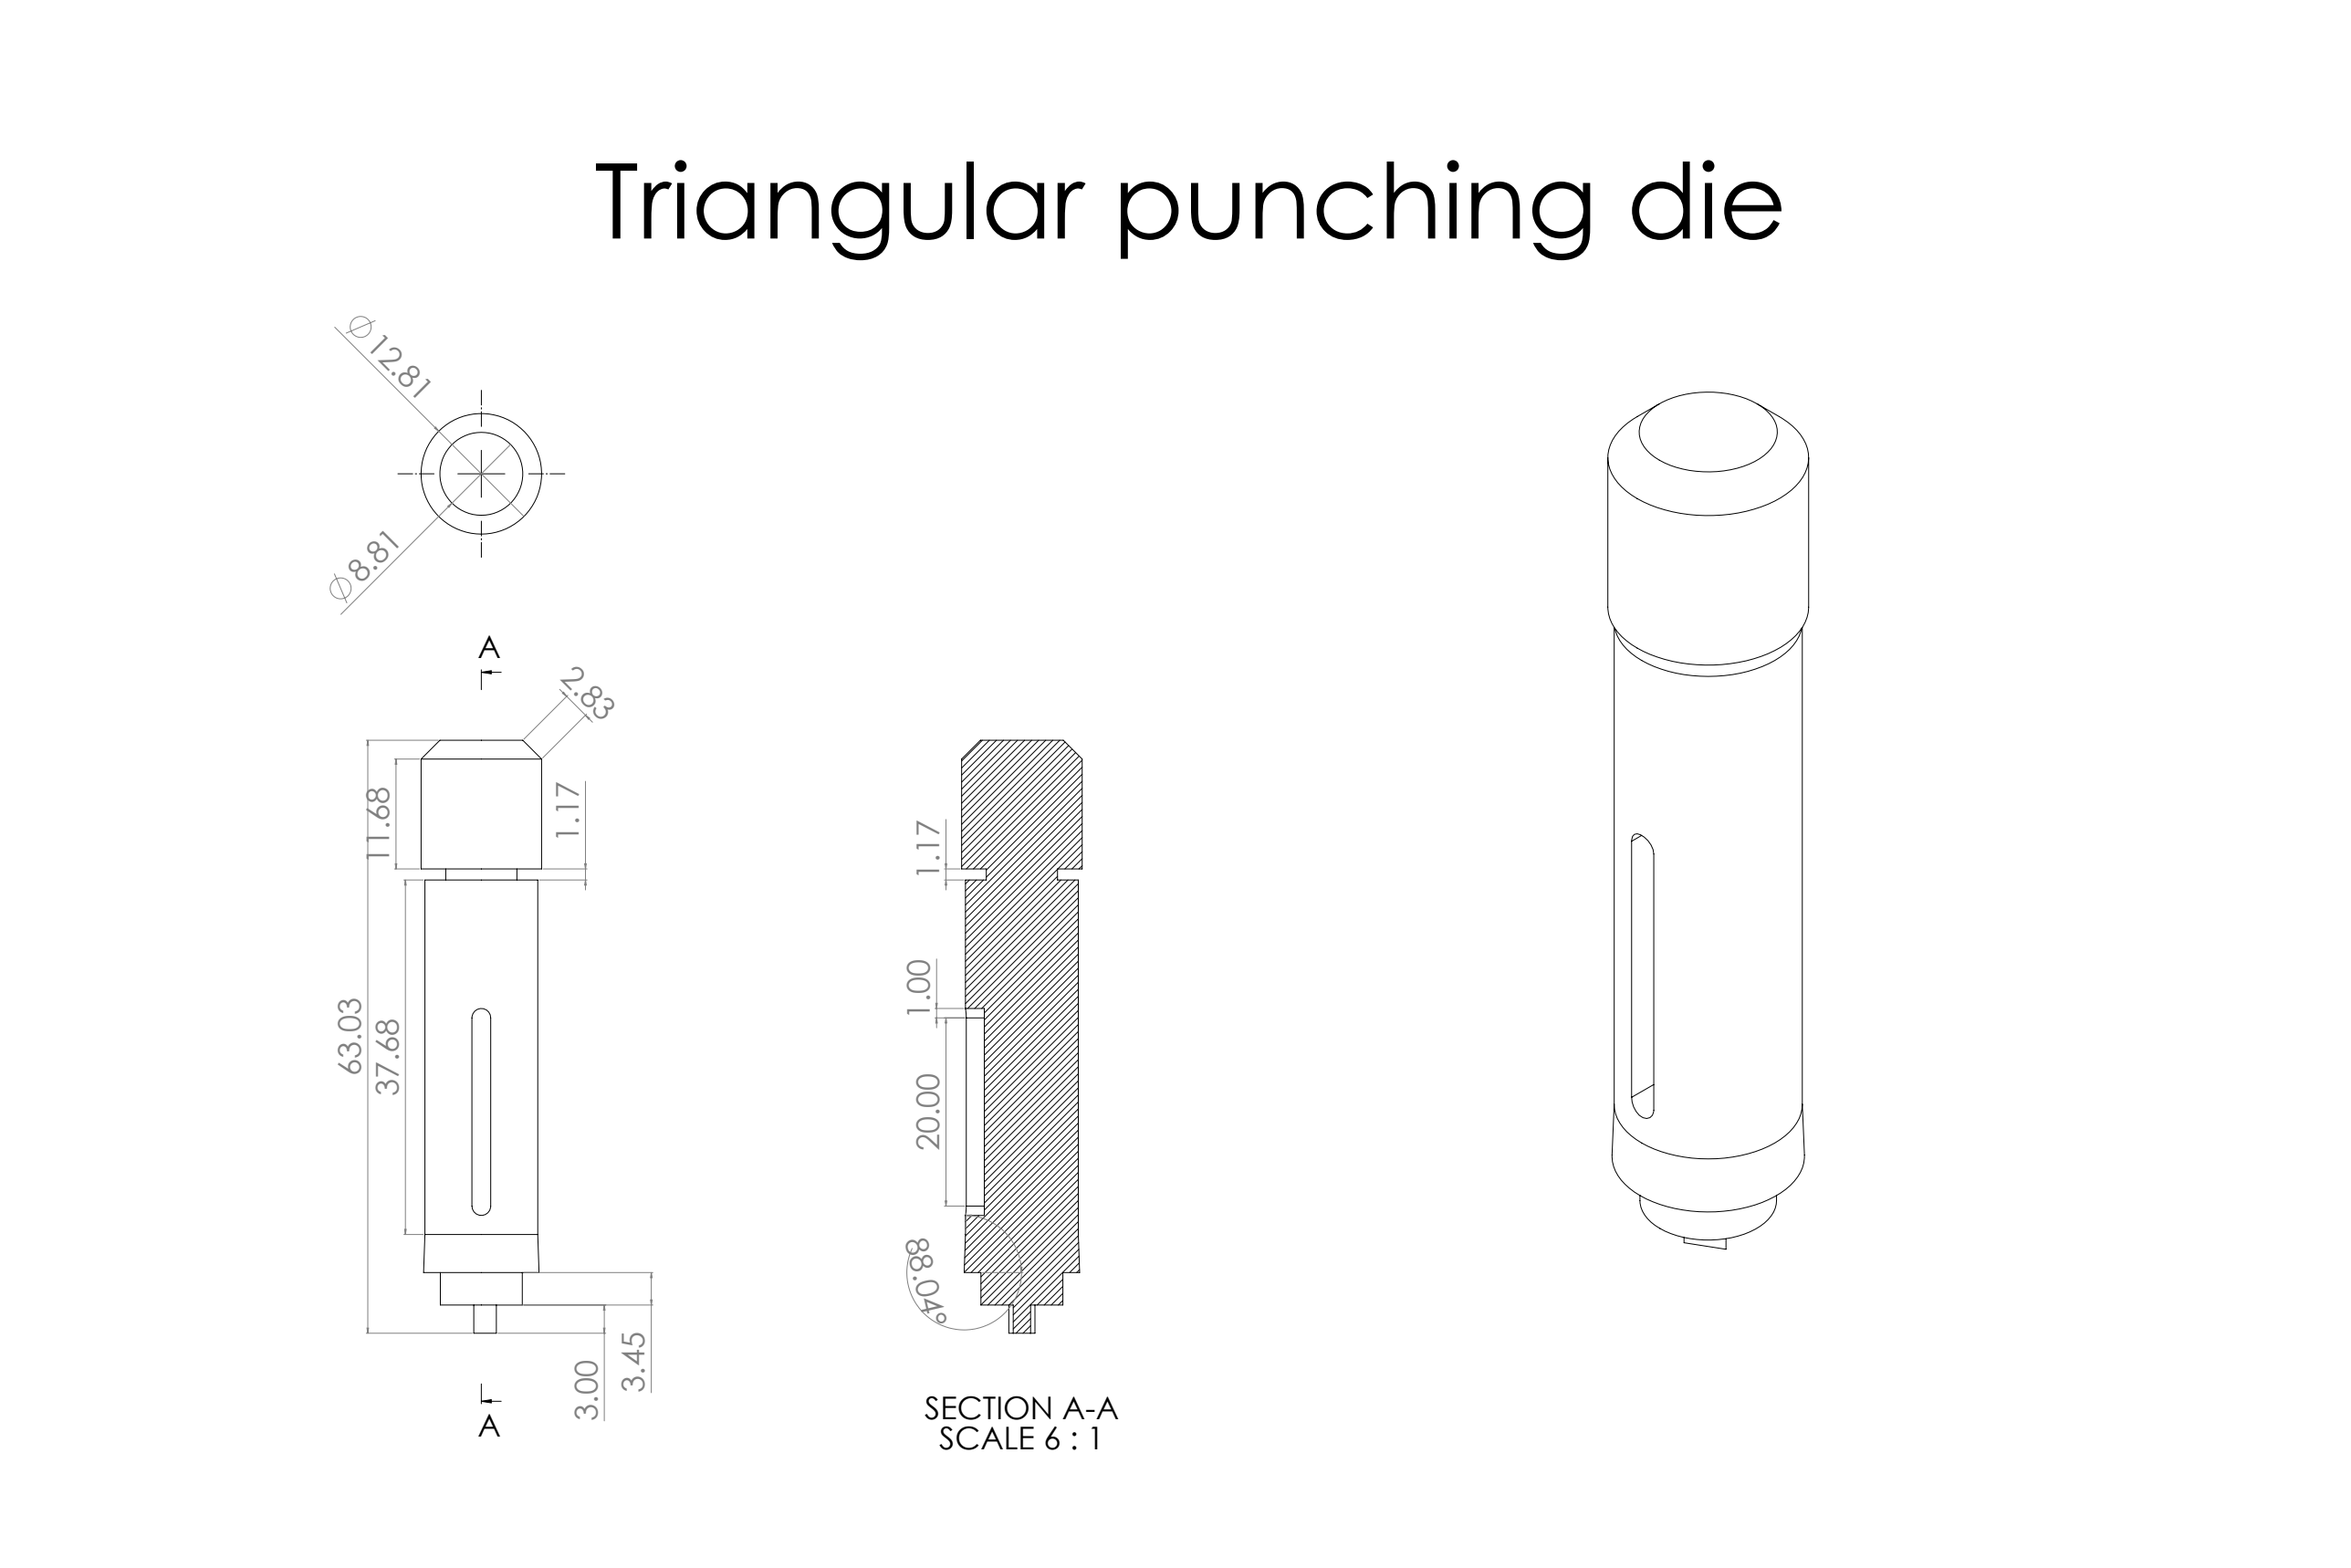
ISO-10303-21;
HEADER;
FILE_DESCRIPTION (('STEP AP214'),
    '1' );
FILE_NAME ('Triangular punching die.step',
    '2026-10-24T22:54:28',
    ( '' ),
    ( '' ),
    'SwSTEP 2.0',
    'SolidWorks 2025',
    '' );
FILE_SCHEMA (( 'AUTOMOTIVE_DESIGN' ));
ENDSEC;

DATA;
#6=DIRECTION ( 'NONE',  ( 0.000000000000000000, -1.000000000000000000, 0.000000000000000000 ) ) ;
#9=CARTESIAN_POINT ( 'NONE',  ( -69.92837670882107659, -20.78299143688747819, 3.916079783099623679 ) ) ;
#20=ORIENTED_EDGE ( 'NONE', *, *, #32884, .T. ) ;
#72=DIRECTION ( 'NONE',  ( -0.000000000000000000, 1.000000000000000000, -0.000000000000000000 ) ) ;
#76=EDGE_CURVE ( 'NONE', #14380, #23841, #36922, .T. ) ;
#84=DIRECTION ( 'NONE',  ( 0.8660254037844393737, 0.000000000000000000, 0.4999999999999985567 ) ) ;
#98=ORIENTED_EDGE ( 'NONE', *, *, #35067, .F. ) ;
#125=EDGE_CURVE ( 'NONE', #38679, #29790, #4804, .T. ) ;
#202=ORIENTED_EDGE ( 'NONE', *, *, #26812, .F. ) ;
#306=ORIENTED_EDGE ( 'NONE', *, *, #22254, .F. ) ;
#395=CIRCLE ( 'NONE', #29328, 6.406751979251626317 ) ;
#462=VERTEX_POINT ( 'NONE', #32769 ) ;
#473=CARTESIAN_POINT ( 'NONE',  ( -70.92837670882107659, 26.72470171467712063, 0.000000000000000000 ) ) ;
#571=ADVANCED_FACE ( 'NONE', ( #22696 ), #35460, .T. ) ;
#611=CARTESIAN_POINT ( 'NONE',  ( -71.90198294515647603, -0.5205283187954542479, 5.920697336060230853 ) ) ;
#644=FACE_OUTER_BOUND ( 'NONE', #40034, .T. ) ;
#810=LINE ( 'NONE', #13343, #16776 ) ;
#853=CARTESIAN_POINT ( 'NONE',  ( -70.92837670882107659, -27.85319909218681644, 0.000000000000000000 ) ) ;
#900=ORIENTED_EDGE ( 'NONE', *, *, #14039, .T. ) ;
#923=FACE_BOUND ( 'NONE', #15811, .T. ) ;
#955=CIRCLE ( 'NONE', #2272, 6.406751979251626317 ) ;
#962=ORIENTED_EDGE ( 'NONE', *, *, #2526, .F. ) ;
#1010=VERTEX_POINT ( 'NONE', #1619 ) ;
#1197=CARTESIAN_POINT ( 'NONE',  ( -71.72837670882105954, -31.30579396504363388, -1.385640646055078307 ) ) ;
#1304=ORIENTED_EDGE ( 'NONE', *, *, #8540, .T. ) ;
#1306=CARTESIAN_POINT ( 'NONE',  ( -70.39213229241123315, 0.06107131307206801335, 5.988032920670404380 ) ) ;
#1331=ADVANCED_FACE ( 'NONE', ( #20901 ), #9845, .T. ) ;
#1414=CARTESIAN_POINT ( 'NONE',  ( -71.78177034180626492, -21.31587262608876543, 5.951446729975963912 ) ) ;
#1470=DIRECTION ( 'NONE',  ( 0.000000000000000000, 0.000000000000000000, 1.000000000000000000 ) ) ;
#1495=CARTESIAN_POINT ( 'NONE',  ( -70.92837670882107659, 28.72470171467712063, 0.000000000000000000 ) ) ;
#1568=DIRECTION ( 'NONE',  ( -0.000000000000000000, 1.000000000000000000, -0.000000000000000000 ) ) ;
#1574=EDGE_LOOP ( 'NONE', ( #33274, #14393, #25939, #14553 ) ) ;
#1583=LINE ( 'NONE', #1197, #20933 ) ;
#1607=CARTESIAN_POINT ( 'NONE',  ( -71.92837670882107659, -20.78299143688747819, 5.928123921495630277 ) ) ;
#1615=EDGE_LOOP ( 'NONE', ( #22756, #962 ) ) ;
#1619=CARTESIAN_POINT ( 'NONE',  ( -70.92837670882107659, 28.72470171467712063, -4.406751979251624540 ) ) ;
#1643=CYLINDRICAL_SURFACE ( 'NONE', #6437, 6.406751979251626317 ) ;
#1676=CARTESIAN_POINT ( 'NONE',  ( -70.92837670882074974, 0.2169278855384722815, 6.000000000000007994 ) ) ;
#1704=CARTESIAN_POINT ( 'NONE',  ( -70.70332177653823180, 0.1913546399533780362, 3.995777704139396924 ) ) ;
#1788=DIRECTION ( 'NONE',  ( 0.8660254037844393737, 0.000000000000000000, 0.4999999999999985567 ) ) ;
#1814=CARTESIAN_POINT ( 'NONE',  ( -71.46462112523092003, -21.62705418684702252, 5.988032920670398163 ) ) ;
#1828=CARTESIAN_POINT ( 'NONE',  ( -70.42442292110172275, -21.65671257467926836, 5.980030958859729573 ) ) ;
#1962=DIRECTION ( 'NONE',  ( 1.000000000000000000, 0.000000000000000000, 0.000000000000000000 ) ) ;
#1987=ADVANCED_FACE ( 'NONE', ( #2899 ), #14440, .T. ) ;
#2112=CARTESIAN_POINT ( 'NONE',  ( -70.21272673770054951, -0.07566977545864603250, 3.957576123060443596 ) ) ;
#2119=CARTESIAN_POINT ( 'NONE',  ( -71.90228189594579078, -21.04538751579064737, 5.920650877785229582 ) ) ;
#2218=CARTESIAN_POINT ( 'NONE',  ( -69.92837670882107659, -20.78299143688747819, 5.928123921495640936 ) ) ;
#2272=AXIS2_PLACEMENT_3D ( 'NONE', #11107, #29658, #1470 ) ;
#2282=VERTEX_POINT ( 'NONE', #23335 ) ;
#2314=CARTESIAN_POINT ( 'NONE',  ( -71.70854571598145810, -0.1474806467180565794, 5.961650403247826802 ) ) ;
#2318=AXIS2_PLACEMENT_3D ( 'NONE', #30036, #14373, #26943 ) ;
#2319=ORIENTED_EDGE ( 'NONE', *, *, #33578, .T. ) ;
#2323=CARTESIAN_POINT ( 'NONE',  ( -71.54295603092448630, -21.58232592843834396, 5.969163363928941202 ) ) ;
#2365=DIRECTION ( 'NONE',  ( -0.000000000000000000, 1.000000000000000000, 0.000000000000000000 ) ) ;
#2370=CIRCLE ( 'NONE', #36523, 6.000000000000005329 ) ;
#2436=CARTESIAN_POINT ( 'NONE',  ( -70.30712919725708332, -21.57437711518543111, 5.980324962551068602 ) ) ;
#2496=CARTESIAN_POINT ( 'NONE',  ( -71.45033707005815415, -21.67496598542010489, 3.980161455544446891 ) ) ;
#2526=EDGE_CURVE ( 'NONE', #5538, #38785, #4624, .T. ) ;
#2543=ORIENTED_EDGE ( 'NONE', *, *, #24789, .T. ) ;
#2557=AXIS2_PLACEMENT_3D ( 'NONE', #15181, #27740, #40293 ) ;
#2563=LINE ( 'NONE', #40201, #30748 ) ;
#2576=CIRCLE ( 'NONE', #38044, 4.357836081054403010 ) ;
#2617=CARTESIAN_POINT ( 'NONE',  ( -70.92837670882107659, -31.30579396504363388, 0.000000000000000000 ) ) ;
#2622=EDGE_CURVE ( 'NONE', #23841, #33142, #10877, .T. ) ;
#2731=CARTESIAN_POINT ( 'NONE',  ( -71.92837670882107659, -0.7434385580723641418, 3.916079783099621014 ) ) ;
#2824=VECTOR ( 'NONE', #17716, 1000.000000000000000 ) ;
#2844=CARTESIAN_POINT ( 'NONE',  ( -71.15343164110390717, -21.75733751372833069, 6.007821842535416401 ) ) ;
#2862=EDGE_CURVE ( 'NONE', #1010, #27757, #28317, .T. ) ;
#2899=FACE_OUTER_BOUND ( 'NONE', #9131, .T. ) ;
#2934=B_SPLINE_CURVE_WITH_KNOTS ( 'NONE', 3,
 ( #8373, #17839, #39671, #1828, #26919, #27121, #5304, #39463, #11454, #23815 ),
 .UNSPECIFIED., .F., .F.,
 ( 4, 2, 2, 2, 4 ),
 ( 0.001566344281586717164, 0.001957551653609773592, 0.002348759025632830236, 0.002739966397655886447, 0.003131173769678943092 ),
 .UNSPECIFIED. ) ;
#2950=DIRECTION ( 'NONE',  ( -0.000000000000000000, 1.000000000000000000, -0.000000000000000000 ) ) ;
#3016=VECTOR ( 'NONE', #6358, 1000.000000000000000 ) ;
#3038=CARTESIAN_POINT ( 'NONE',  ( -69.95453796102918886, -0.5206348589351952327, 3.920659437262051128 ) ) ;
#3059=CARTESIAN_POINT ( 'NONE',  ( -71.26311553261176357, -21.73200267494512161, 3.991660656778087901 ) ) ;
#3150=CARTESIAN_POINT ( 'NONE',  ( -70.92661119047551210, 0.2232129446074198609, 6.013069300985390164 ) ) ;
#3160=FACE_OUTER_BOUND ( 'NONE', #26573, .T. ) ;
#3178=ORIENTED_EDGE ( 'NONE', *, *, #7572, .F. ) ;
#3212=ADVANCED_FACE ( 'NONE', ( #20406 ), #22912, .F. ) ;
#3215=CYLINDRICAL_SURFACE ( 'NONE', #32680, 6.000000000000005329 ) ;
#3394=CARTESIAN_POINT ( 'NONE',  ( -71.92837670882107659, -0.7829914368874776320, 3.916079783099624567 ) ) ;
#3430=CARTESIAN_POINT ( 'NONE',  ( -70.92837670882107659, -27.85319909218681644, 0.000000000000000000 ) ) ;
#3553=DIRECTION ( 'NONE',  ( 1.000000000000000000, 0.000000000000000000, 0.000000000000000000 ) ) ;
#3556=VERTEX_POINT ( 'NONE', #37877 ) ;
#3634=AXIS2_PLACEMENT_3D ( 'NONE', #8388, #17438, #33545 ) ;
#3739=DIRECTION ( 'NONE',  ( 0.000000000000000000, 0.000000000000000000, 1.000000000000000000 ) ) ;
#3782=DIRECTION ( 'NONE',  ( 0.000000000000000000, 0.000000000000000000, -1.000000000000000000 ) ) ;
#3794=PLANE ( 'NONE',  #7689 ) ;
#3809=AXIS2_PLACEMENT_3D ( 'NONE', #18051, #21163, #14976 ) ;
#3859=ORIENTED_EDGE ( 'NONE', *, *, #10125, .F. ) ;
#3874=AXIS2_PLACEMENT_3D ( 'NONE', #7544, #7343, #4273 ) ;
#3898=EDGE_CURVE ( 'NONE', #16025, #29790, #6157, .T. ) ;
#3957=VECTOR ( 'NONE', #1568, 1000.000000000000000 ) ;
#3959=B_SPLINE_CURVE_WITH_KNOTS ( 'NONE', 3,
 ( #34198, #37249, #8629, #33779, #5557, #2496, #33990, #24286 ),
 .UNSPECIFIED., .F., .F.,
 ( 4, 2, 2, 4 ),
 ( 0.000000000000000000, 0.1250305178534004968, 0.2500610357068009937, 0.5001220714135948819 ),
 .UNSPECIFIED. ) ;
#3972=CARTESIAN_POINT ( 'NONE',  ( -70.12941285977503014, -0.1676659666690925865, 5.947291465561957757 ) ) ;
#4011=VERTEX_POINT ( 'NONE', #4097 ) ;
#4055=SHAPE_DEFINITION_REPRESENTATION ( #35129, #39290 ) ;
#4058=EDGE_CURVE ( 'NONE', #25957, #16025, #11437, .T. ) ;
#4097=CARTESIAN_POINT ( 'NONE',  ( -70.92837670882107659, -23.80776546975053165, 6.000000000000005329 ) ) ;
#4138=ORIENTED_EDGE ( 'NONE', *, *, #11281, .F. ) ;
#4201=CARTESIAN_POINT ( 'NONE',  ( -71.72837670882105954, -34.30579396504363388, 1.385640646055090519 ) ) ;
#4229=PRODUCT ( 'Triangular punching die', 'Triangular punching die', '', ( #32256 ) ) ;
#4233=PLANE ( 'NONE',  #15168 ) ;
#4273=DIRECTION ( 'NONE',  ( 0.000000000000000000, 0.000000000000000000, 1.000000000000000000 ) ) ;
#4395=CARTESIAN_POINT ( 'NONE',  ( -69.92837670882107659, -0.6719362264620037939, 5.928123921495636495 ) ) ;
#4483=CARTESIAN_POINT ( 'NONE',  ( 0.000000000000000000, -34.30579396504363388, 0.000000000000000000 ) ) ;
#4501=CARTESIAN_POINT ( 'NONE',  ( -71.90933819610624766, -21.00662979218648374, 3.919381273429904056 ) ) ;
#4624=CIRCLE ( 'NONE', #20378, 6.138794830819693793 ) ;
#4660=EDGE_CURVE ( 'NONE', #5702, #13186, #26402, .T. ) ;
#4688=CARTESIAN_POINT ( 'NONE',  ( -71.64402667994158946, -21.49031309831630665, 5.969620261456463517 ) ) ;
#4775=CARTESIAN_POINT ( 'NONE',  ( -70.14355411941724583, -0.1632709328201389365, 5.960493810635122180 ) ) ;
#4804=B_SPLINE_CURVE_WITH_KNOTS ( 'NONE', 3,
 ( #11778, #5840, #36316, #5020, #14672, #36713, #8496, #6456, #34681, #3394 ),
 .UNSPECIFIED., .F., .F.,
 ( 4, 2, 2, 2, 4 ),
 ( 0.5001220714136037637, 0.6250915535602028505, 0.7500610357068019374, 0.8750305178534010242, 1.000000000000000000 ),
 .UNSPECIFIED. ) ;
#4915=FACE_OUTER_BOUND ( 'NONE', #7970, .T. ) ;
#4923=VERTEX_POINT ( 'NONE', #39919 ) ;
#4937=( LENGTH_UNIT ( ) NAMED_UNIT ( * ) SI_UNIT ( .MILLI., .METRE. ) );
#5016=AXIS2_PLACEMENT_3D ( 'NONE', #35112, #28916, #32018 ) ;
#5020=CARTESIAN_POINT ( 'NONE',  ( -71.43157283993535600, 0.09103159405784894131, 3.980077070333584821 ) ) ;
#5066=DIRECTION ( 'NONE',  ( 0.000000000000000000, 0.000000000000000000, 1.000000000000000000 ) ) ;
#5088=CARTESIAN_POINT ( 'NONE',  ( -71.83651116356016075, -21.21610000639230975, 3.930990725878106495 ) ) ;
#5098=VECTOR ( 'NONE', #39151, 1000.000000000000000 ) ;
#5170=EDGE_CURVE ( 'NONE', #10250, #36751, #27655, .T. ) ;
#5227=PLANE ( 'NONE',  #5811 ) ;
#5275=ORIENTED_EDGE ( 'NONE', *, *, #7116, .F. ) ;
#5281=ORIENTED_EDGE ( 'NONE', *, *, #38674, .T. ) ;
#5304=CARTESIAN_POINT ( 'NONE',  ( -70.05487543777402948, -21.28726014413347656, 5.936291904728155266 ) ) ;
#5317=VERTEX_POINT ( 'NONE', #21005 ) ;
#5385=CARTESIAN_POINT ( 'NONE',  ( -71.92602134074772380, -0.7038144147489171498, 3.916479336966925295 ) ) ;
#5426=DIRECTION ( 'NONE',  ( -0.000000000000000000, 1.000000000000000000, -0.000000000000000000 ) ) ;
#5476=CARTESIAN_POINT ( 'NONE',  ( -69.32837670882108227, -31.30579396504363388, 1.870248747537495149E-15 ) ) ;
#5493=CARTESIAN_POINT ( 'NONE',  ( -70.03118149891237465, -21.22462562410226994, 5.944584973090443647 ) ) ;
#5538=VERTEX_POINT ( 'NONE', #40533 ) ;
#5557=CARTESIAN_POINT ( 'NONE',  ( -71.72810306468316810, -21.39745238146776884, 3.947195235487914289 ) ) ;
#5702=VERTEX_POINT ( 'NONE', #29808 ) ;
#5703=CARTESIAN_POINT ( 'NONE',  ( -69.92837670882107659, -20.82254431570259001, 5.928123921495640936 ) ) ;
#5710=VERTEX_POINT ( 'NONE', #16834 ) ;
#5712=AXIS2_PLACEMENT_3D ( 'NONE', #30670, #9024, #24268 ) ;
#5807=CARTESIAN_POINT ( 'NONE',  ( -71.92837670882107659, -20.78299143688747819, 5.916079783099621459 ) ) ;
#5811=AXIS2_PLACEMENT_3D ( 'NONE', #18177, #2365, #9122 ) ;
#5840=CARTESIAN_POINT ( 'NONE',  ( -71.06003735762037365, 0.2170295740194823630, 3.999999999923639304 ) ) ;
#5870=EDGE_LOOP ( 'NONE', ( #27582, #40559, #22660, #20284 ) ) ;
#5893=DIRECTION ( 'NONE',  ( 4.199171463528975886E-18, -0.9994119649315837961, 0.03428883712799970368 ) ) ;
#5988=EDGE_LOOP ( 'NONE', ( #30833, #13755, #27770, #37888 ) ) ;
#6023=DIRECTION ( 'NONE',  ( -0.000000000000000000, 1.000000000000000000, -0.000000000000000000 ) ) ;
#6116=CARTESIAN_POINT ( 'NONE',  ( -70.81922763566456069, -21.77701682883130019, 6.011051262898291725 ) ) ;
#6142=EDGE_CURVE ( 'NONE', #4923, #5702, #21778, .T. ) ;
#6157=LINE ( 'NONE', #31279, #12541 ) ;
#6271=ORIENTED_EDGE ( 'NONE', *, *, #11072, .T. ) ;
#6358=DIRECTION ( 'NONE',  ( 0.000000000000000000, 0.000000000000000000, -1.000000000000000000 ) ) ;
#6427=CARTESIAN_POINT ( 'NONE',  ( -70.31344945295795412, -21.58221595790078950, 3.969121680884525105 ) ) ;
#6437=AXIS2_PLACEMENT_3D ( 'NONE', #10485, #14181, #23065 ) ;
#6456=CARTESIAN_POINT ( 'NONE',  ( -71.90176653367559823, -0.5198039855910460139, 3.920732911925276287 ) ) ;
#6490=ORIENTED_EDGE ( 'NONE', *, *, #4660, .F. ) ;
#6630=EDGE_CURVE ( 'NONE', #38785, #5538, #36078, .T. ) ;
#6719=EDGE_CURVE ( 'NONE', #39731, #33142, #10570, .T. ) ;
#6822=DIRECTION ( 'NONE',  ( -0.000000000000000000, 1.000000000000000000, -0.000000000000000000 ) ) ;
#6930=LINE ( 'NONE', #11967, #25648 ) ;
#6931=ORIENTED_EDGE ( 'NONE', *, *, #33578, .F. ) ;
#6990=VERTEX_POINT ( 'NONE', #25378 ) ;
#7031=CARTESIAN_POINT ( 'NONE',  ( -70.05520034786580652, -0.2785546670064985575, 5.936342406970505969 ) ) ;
#7083=VERTEX_POINT ( 'NONE', #36807 ) ;
#7111=CARTESIAN_POINT ( 'NONE',  ( -70.92837670882107659, 28.72470171467712063, 6.000000000000005329 ) ) ;
#7116=EDGE_CURVE ( 'NONE', #6990, #34705, #20268, .T. ) ;
#7126=ORIENTED_EDGE ( 'NONE', *, *, #39294, .T. ) ;
#7232=CARTESIAN_POINT ( 'NONE',  ( -70.92837670882107659, 28.72470171467712063, -2.000000000000000000 ) ) ;
#7233=CARTESIAN_POINT ( 'NONE',  ( -69.92837670882107659, -0.6505659821428084744, 5.916079783099619682 ) ) ;
#7254=DIRECTION ( 'NONE',  ( 0.000000000000000000, 0.000000000000000000, 1.000000000000000000 ) ) ;
#7276=ORIENTED_EDGE ( 'NONE', *, *, #11043, .T. ) ;
#7343=DIRECTION ( 'NONE',  ( -0.000000000000000000, 1.000000000000000000, -0.000000000000000000 ) ) ;
#7357=B_SPLINE_CURVE_WITH_KNOTS ( 'NONE', 3,
 ( #8551, #8957, #3038, #14721, #24414, #34122, #18021, #11630 ),
 .UNSPECIFIED., .F., .F.,
 ( 4, 2, 2, 4 ),
 ( 0.000000000000000000, 0.1250305178534032724, 0.2500610357068065448, 0.5001220714136037637 ),
 .UNSPECIFIED. ) ;
#7367=CARTESIAN_POINT ( 'NONE',  ( -71.26311553261176357, -21.73200267494512161, 6.003704795174108710 ) ) ;
#7423=CARTESIAN_POINT ( 'NONE',  ( -69.92837670882107659, -20.78299143688747819, 5.916079783099620570 ) ) ;
#7434=FACE_BOUND ( 'NONE', #33299, .T. ) ;
#7486=FACE_OUTER_BOUND ( 'NONE', #22537, .T. ) ;
#7509=CIRCLE ( 'NONE', #35800, 4.406751979251624540 ) ;
#7544=CARTESIAN_POINT ( 'NONE',  ( -70.92837670882107659, -23.80776546975053165, 0.000000000000000000 ) ) ;
#7567=ORIENTED_EDGE ( 'NONE', *, *, #24444, .F. ) ;
#7572=EDGE_CURVE ( 'NONE', #10043, #14380, #28058, .T. ) ;
#7634=CARTESIAN_POINT ( 'NONE',  ( -69.92837670882107659, -0.7829914368874778541, 5.916079783099621459 ) ) ;
#7689=AXIS2_PLACEMENT_3D ( 'NONE', #16316, #32392, #28886 ) ;
#7767=AXIS2_PLACEMENT_3D ( 'NONE', #2617, #40052, #15341 ) ;
#7769=CARTESIAN_POINT ( 'NONE',  ( -71.78177034180626492, -21.31587262608876543, 3.939402591579943547 ) ) ;
#7809=AXIS2_PLACEMENT_3D ( 'NONE', #7232, #20184, #9916 ) ;
#7842=CARTESIAN_POINT ( 'NONE',  ( -64.92837670882106238, 13.87661300689593880, 0.000000000000000000 ) ) ;
#7858=DIRECTION ( 'NONE',  ( -0.000000000000000000, 1.000000000000000000, -0.000000000000000000 ) ) ;
#7874=CARTESIAN_POINT ( 'NONE',  ( -69.32837670882108227, -34.30579396504363388, 1.870248747537495149E-15 ) ) ;
#7970=EDGE_LOOP ( 'NONE', ( #19165, #8346, #10889, #5275 ) ) ;
#8049=FACE_OUTER_BOUND ( 'NONE', #12714, .T. ) ;
#8074=EDGE_CURVE ( 'NONE', #1010, #8622, #31565, .T. ) ;
#8105=EDGE_CURVE ( 'NONE', #34705, #6990, #32880, .T. ) ;
#8259=EDGE_LOOP ( 'NONE', ( #36223, #39781, #8815, #24678 ) ) ;
#8310=VECTOR ( 'NONE', #30487, 1000.000000000000000 ) ;
#8346=ORIENTED_EDGE ( 'NONE', *, *, #10125, .T. ) ;
#8350=EDGE_LOOP ( 'NONE', ( #10985, #31039, #38270 ) ) ;
#8373=CARTESIAN_POINT ( 'NONE',  ( -70.92837670882140344, -21.78291075931342391, 6.000000000000002665 ) ) ;
#8388=CARTESIAN_POINT ( 'NONE',  ( -71.72837670882105954, -34.30579396504363388, -1.385640646055078307 ) ) ;
#8390=DIRECTION ( 'NONE',  ( 0.000000000000000000, 0.000000000000000000, 1.000000000000000000 ) ) ;
#8440=VERTEX_POINT ( 'NONE', #38010 ) ;
#8448=DIRECTION ( 'NONE',  ( 0.000000000000000000, -1.000000000000000000, 0.000000000000000000 ) ) ;
#8454=CARTESIAN_POINT ( 'NONE',  ( -71.25654746924473670, 0.1680418597759353594, 6.003896035474988402 ) ) ;
#8496=CARTESIAN_POINT ( 'NONE',  ( -71.80166262301922586, -0.2784082907551633790, 3.936323582618165950 ) ) ;
#8540=EDGE_CURVE ( 'NONE', #39825, #5317, #6930, .T. ) ;
#8551=CARTESIAN_POINT ( 'NONE',  ( -69.92837670882107659, -0.7829914368874778541, 3.916079783099621014 ) ) ;
#8568=CARTESIAN_POINT ( 'NONE',  ( -70.70940173728274658, -21.76495738335424690, 6.009053033063224802 ) ) ;
#8570=EDGE_CURVE ( 'NONE', #23332, #27757, #40379, .T. ) ;
#8586=LINE ( 'NONE', #9350, #31786 ) ;
#8606=AXIS2_PLACEMENT_3D ( 'NONE', #34871, #72, #30754 ) ;
#8622=VERTEX_POINT ( 'NONE', #36346 ) ;
#8629=CARTESIAN_POINT ( 'NONE',  ( -71.90221545680498139, -21.04534801433412028, 3.920659437232132394 ) ) ;
#8647=DIRECTION ( 'NONE',  ( 0.000000000000000000, 0.000000000000000000, 1.000000000000000000 ) ) ;
#8659=CARTESIAN_POINT ( 'NONE',  ( -71.62860729996657483, -0.06907469158448548141, 3.958999674376896039 ) ) ;
#8666=CARTESIAN_POINT ( 'NONE',  ( -71.92837670882107659, -20.78299143688747819, 5.916079783099621459 ) ) ;
#8721=CARTESIAN_POINT ( 'NONE',  ( -69.92837670882107659, -20.78299143688747819, 5.916079783099621459 ) ) ;
#8764=ORIENTED_EDGE ( 'NONE', *, *, #11281, .T. ) ;
#8768=CARTESIAN_POINT ( 'NONE',  ( -69.93541594206888590, -20.90143516061696616, 3.917265324091089518 ) ) ;
#8815=ORIENTED_EDGE ( 'NONE', *, *, #25812, .F. ) ;
#8901=DIRECTION ( 'NONE',  ( -0.000000000000000000, 1.000000000000000000, -0.000000000000000000 ) ) ;
#8941=AXIS2_PLACEMENT_3D ( 'NONE', #21020, #39951, #8647 ) ;
#8957=CARTESIAN_POINT ( 'NONE',  ( -69.92844875602597199, -0.6521111472992819902, 3.916091961299970059 ) ) ;
#8958=CARTESIAN_POINT ( 'NONE',  ( -70.92837670882107659, 28.72470171467712063, 0.000000000000000000 ) ) ;
#8978=CARTESIAN_POINT ( 'NONE',  ( -70.14820770166069508, -21.41850222705690143, 3.949606264851799775 ) ) ;
#9024=DIRECTION ( 'NONE',  ( -0.000000000000000000, 1.000000000000000000, -0.000000000000000000 ) ) ;
#9057=ORIENTED_EDGE ( 'NONE', *, *, #40617, .T. ) ;
#9075=CARTESIAN_POINT ( 'NONE',  ( -71.82557191872977853, -0.3413572496726843264, 3.932540834694423726 ) ) ;
#9082=CARTESIAN_POINT ( 'NONE',  ( -71.92837670882107659, -20.91541689163215523, 5.916079783099619682 ) ) ;
#9091=CIRCLE ( 'NONE', #7767, 4.357836081054403010 ) ;
#9122=DIRECTION ( 'NONE',  ( 0.000000000000000000, 0.000000000000000000, 1.000000000000000000 ) ) ;
#9131=EDGE_LOOP ( 'NONE', ( #10423, #7126, #11894, #34602 ) ) ;
#9180=DIRECTION ( 'NONE',  ( -0.000000000000000000, 1.000000000000000000, -0.000000000000000000 ) ) ;
#9188=CARTESIAN_POINT ( 'NONE',  ( -70.60020594839741648, -21.73402473355089271, 6.003896035474983073 ) ) ;
#9260=CIRCLE ( 'NONE', #8606, 4.357836081054403010 ) ;
#9274=CARTESIAN_POINT ( 'NONE',  ( -71.62860729996657483, -0.06907469158448548141, 5.971043812772921733 ) ) ;
#9276=EDGE_CURVE ( 'NONE', #36200, #38679, #7357, .T. ) ;
#9302=EDGE_CURVE ( 'NONE', #4011, #5538, #34527, .T. ) ;
#9350=CARTESIAN_POINT ( 'NONE',  ( -70.92837670882107659, 28.72470171467712063, -3.784187430299790211 ) ) ;
#9485=DIRECTION ( 'NONE',  ( 0.000000000000000000, 0.000000000000000000, 1.000000000000000000 ) ) ;
#9569=ORIENTED_EDGE ( 'NONE', *, *, #27926, .F. ) ;
#9618=ADVANCED_FACE ( 'NONE', ( #10587 ), #4233, .F. ) ;
#9648=CIRCLE ( 'NONE', #5712, 3.784187430299790211 ) ;
#9697=B_SPLINE_CURVE_WITH_KNOTS ( 'NONE', 3,
 ( #8666, #9082, #2119, #36886, #27812, #2323, #21245, #21660, #40365, #18139 ),
 .UNSPECIFIED., .F., .F.,
 ( 4, 2, 2, 2, 4 ),
 ( 0.000000000000000000, 0.0003915860703966792910, 0.0007831721407933585821, 0.001174758211190037819, 0.001566344281586717164 ),
 .UNSPECIFIED. ) ;
#9702=VERTEX_POINT ( 'NONE', #18389 ) ;
#9797=ORIENTED_EDGE ( 'NONE', *, *, #3898, .F. ) ;
#9818=DIRECTION ( 'NONE',  ( -0.000000000000000000, 1.000000000000000000, -0.000000000000000000 ) ) ;
#9845=CONICAL_SURFACE ( 'NONE', #21667, 6.406751979251626317, 0.7853981633974482790 ) ;
#9899=ORIENTED_EDGE ( 'NONE', *, *, #22254, .T. ) ;
#9900=ADVANCED_FACE ( 'NONE', ( #19217 ), #35683, .T. ) ;
#9916=DIRECTION ( 'NONE',  ( 0.000000000000000000, 0.000000000000000000, 1.000000000000000000 ) ) ;
#9921=AXIS2_PLACEMENT_3D ( 'NONE', #24520, #14625, #21233 ) ;
#10043=VERTEX_POINT ( 'NONE', #17307 ) ;
#10114=VECTOR ( 'NONE', #36242, 1000.000000000000000 ) ;
#10125=EDGE_CURVE ( 'NONE', #2282, #8440, #37505, .T. ) ;
#10250=VERTEX_POINT ( 'NONE', #24104 ) ;
#10285=DIRECTION ( 'NONE',  ( -0.000000000000000000, 1.000000000000000000, -0.000000000000000000 ) ) ;
#10327=CARTESIAN_POINT ( 'NONE',  ( -69.92837670882107659, -0.7829914368874777431, 5.916079783099621459 ) ) ;
#10338=DIRECTION ( 'NONE',  ( -0.000000000000000000, 1.000000000000000000, -0.000000000000000000 ) ) ;
#10406=DIRECTION ( 'NONE',  ( 0.000000000000000000, 0.000000000000000000, 1.000000000000000000 ) ) ;
#10423=ORIENTED_EDGE ( 'NONE', *, *, #21751, .F. ) ;
#10453=DIRECTION ( 'NONE',  ( 0.000000000000000000, -0.9994119649315837961, -0.03428883712799970368 ) ) ;
#10485=CARTESIAN_POINT ( 'NONE',  ( -70.92837670882107659, 28.72470171467712063, 0.000000000000000000 ) ) ;
#10499=( NAMED_UNIT ( * ) SI_UNIT ( $, .STERADIAN. ) SOLID_ANGLE_UNIT ( ) );
#10544=ORIENTED_EDGE ( 'NONE', *, *, #6630, .T. ) ;
#10548=LINE ( 'NONE', #13442, #5098 ) ;
#10570=LINE ( 'NONE', #16944, #26860 ) ;
#10587=FACE_OUTER_BOUND ( 'NONE', #26046, .T. ) ;
#10628=ORIENTED_EDGE ( 'NONE', *, *, #30089, .F. ) ;
#10715=DIRECTION ( 'NONE',  ( 0.000000000000000000, -0.000000000000000000, -1.000000000000000000 ) ) ;
#10727=DIRECTION ( 'NONE',  ( 0.000000000000000000, 0.000000000000000000, 1.000000000000000000 ) ) ;
#10748=FACE_OUTER_BOUND ( 'NONE', #5870, .T. ) ;
#10815=EDGE_CURVE ( 'NONE', #40423, #4923, #9260, .T. ) ;
#10823=DIRECTION ( 'NONE',  ( -0.000000000000000000, 1.000000000000000000, -0.000000000000000000 ) ) ;
#10877=LINE ( 'NONE', #5476, #21705 ) ;
#10888=ORIENTED_EDGE ( 'NONE', *, *, #35911, .F. ) ;
#10889=ORIENTED_EDGE ( 'NONE', *, *, #14799, .T. ) ;
#10939=CARTESIAN_POINT ( 'NONE',  ( -70.92837670882107659, 28.72470171467712063, 4.000000000000005329 ) ) ;
#10983=DIRECTION ( 'NONE',  ( 0.000000000000000000, 0.000000000000000000, -1.000000000000000000 ) ) ;
#10985=ORIENTED_EDGE ( 'NONE', *, *, #7572, .T. ) ;
#11000=DIRECTION ( 'NONE',  ( -0.000000000000000000, 1.000000000000000000, -0.000000000000000000 ) ) ;
#11030=CARTESIAN_POINT ( 'NONE',  ( -70.92837670882107659, -23.80776546975053165, 0.000000000000000000 ) ) ;
#11042=CARTESIAN_POINT ( 'NONE',  ( -71.55887904216392315, -21.56717086459383026, 3.967530720604706573 ) ) ;
#11043=EDGE_CURVE ( 'NONE', #3556, #23841, #1583, .T. ) ;
#11054=EDGE_CURVE ( 'NONE', #13186, #5702, #2576, .T. ) ;
#11069=PLANE ( 'NONE',  #3634 ) ;
#11072=EDGE_CURVE ( 'NONE', #4011, #39825, #34110, .T. ) ;
#11107=CARTESIAN_POINT ( 'NONE',  ( -70.92837670882107659, 15.04836564048558500, 0.000000000000000000 ) ) ;
#11114=CARTESIAN_POINT ( 'NONE',  ( -70.92837670882074974, 0.2169278855384722815, 6.000000000000007994 ) ) ;
#11137=CARTESIAN_POINT ( 'NONE',  ( -70.21272673770054951, -0.07566977545864603250, 5.969620261456469734 ) ) ;
#11149=ORIENTED_EDGE ( 'NONE', *, *, #8074, .T. ) ;
#11198=DIRECTION ( 'NONE',  ( 8.659560562354932858E-17, -0.7071067811865474617, 0.7071067811865474617 ) ) ;
#11242=ORIENTED_EDGE ( 'NONE', *, *, #2862, .T. ) ;
#11281=EDGE_CURVE ( 'NONE', #4923, #40423, #9091, .T. ) ;
#11296=ORIENTED_EDGE ( 'NONE', *, *, #32884, .F. ) ;
#11334=CARTESIAN_POINT ( 'NONE',  ( -69.94741522153590552, -0.5593530815884721896, 3.919381273429904944 ) ) ;
#11422=DIRECTION ( 'NONE',  ( -0.000000000000000000, 1.000000000000000000, -0.000000000000000000 ) ) ;
#11434=DIRECTION ( 'NONE',  ( -0.000000000000000000, 1.000000000000000000, -0.000000000000000000 ) ) ;
#11437=LINE ( 'NONE', #27105, #15839 ) ;
#11442=CARTESIAN_POINT ( 'NONE',  ( -71.36981149190343388, -21.68728802194536698, 5.996540489601002832 ) ) ;
#11454=CARTESIAN_POINT ( 'NONE',  ( -69.92837670882109080, -20.91528719346852583, 5.916079783099622347 ) ) ;
#11475=MECHANICAL_DESIGN_GEOMETRIC_PRESENTATION_REPRESENTATION('',(#31237),#12133);
#11533=CIRCLE ( 'NONE', #30618, 6.406751979251626317 ) ;
#11551=ADVANCED_FACE ( 'NONE', ( #29536, #11990 ), #5227, .F. ) ;
#11630=CARTESIAN_POINT ( 'NONE',  ( -70.92837671539291478, 0.2169278822316458022, 3.999987187540717137 ) ) ;
#11647=CARTESIAN_POINT ( 'NONE',  ( -71.04476776058896803, -21.78243674987466605, 3.999856464806923473 ) ) ;
#11721=EDGE_LOOP ( 'NONE', ( #19383, #15515, #12945, #31925 ) ) ;
#11737=CARTESIAN_POINT ( 'NONE',  ( -71.35621909400492768, 0.1208619214844364048, 5.996770606117012292 ) ) ;
#11778=CARTESIAN_POINT ( 'NONE',  ( -70.92837671539291478, 0.2169278822316458022, 3.999987187540717137 ) ) ;
#11825=APPLICATION_CONTEXT ( 'automotive_design' ) ;
#11832=EDGE_CURVE ( 'NONE', #36751, #462, #26262, .T. ) ;
#11856=CARTESIAN_POINT ( 'NONE',  ( -70.93014222716664108, -21.78919581838237463, 4.001025162589363582 ) ) ;
#11894=ORIENTED_EDGE ( 'NONE', *, *, #35615, .T. ) ;
#11921=ORIENTED_EDGE ( 'NONE', *, *, #9276, .T. ) ;
#11947=CARTESIAN_POINT ( 'NONE',  ( -71.14735168035940660, 0.1989745095792901375, 3.997008894667205769 ) ) ;
#11950=ORIENTED_EDGE ( 'NONE', *, *, #33196, .F. ) ;
#11967=CARTESIAN_POINT ( 'NONE',  ( -70.92837670882107659, 28.72470171467712063, -6.000000000000005329 ) ) ;
#11990=FACE_BOUND ( 'NONE', #21791, .T. ) ;
#12133=( GEOMETRIC_REPRESENTATION_CONTEXT ( 3 ) GLOBAL_UNCERTAINTY_ASSIGNED_CONTEXT ( ( #37395 ) ) GLOBAL_UNIT_ASSIGNED_CONTEXT ( ( #23354, #25840, #32429 ) ) REPRESENTATION_CONTEXT ( 'NONE', 'WORKASPACE' ) );
#12166=ADVANCED_FACE ( 'NONE', ( #27197 ), #39755, .F. ) ;
#12327=MANIFOLD_SOLID_BREP ( 'Boss-Extrude8', #12401 ) ;
#12401=CLOSED_SHELL ( 'NONE', ( #39691, #1987, #25949, #21027, #39842, #35251, #13945, #36039, #9900, #12166, #13085, #28260, #37481, #27739, #13394, #11551, #29530, #1331, #38039, #26954, #37778, #38983, #571, #20533, #3212, #9618, #37540 ) ) ;
#12541=VECTOR ( 'NONE', #28168, 1000.000000000000000 ) ;
#12676=CARTESIAN_POINT ( 'NONE',  ( -70.92837670882107659, 28.72470171467712063, 0.000000000000000000 ) ) ;
#12714=EDGE_LOOP ( 'NONE', ( #37433, #13169, #24068, #21564, #13752, #13002 ) ) ;
#12720=DIRECTION ( 'NONE',  ( 0.000000000000000000, 0.000000000000000000, -1.000000000000000000 ) ) ;
#12721=LINE ( 'NONE', #37423, #3016 ) ;
#12737=CARTESIAN_POINT ( 'NONE',  ( -71.80187797986816634, -0.2787227296414631073, 5.936291904728147273 ) ) ;
#12767=ORIENTED_EDGE ( 'NONE', *, *, #4660, .T. ) ;
#12945=ORIENTED_EDGE ( 'NONE', *, *, #26812, .T. ) ;
#13002=ORIENTED_EDGE ( 'NONE', *, *, #125, .F. ) ;
#13052=AXIS2_PLACEMENT_3D ( 'NONE', #3430, #15942, #34919 ) ;
#13085=ADVANCED_FACE ( 'NONE', ( #644 ), #35029, .T. ) ;
#13169=ORIENTED_EDGE ( 'NONE', *, *, #35846, .F. ) ;
#13186=VERTEX_POINT ( 'NONE', #13788 ) ;
#13211=AXIS2_PLACEMENT_3D ( 'NONE', #1495, #7858, #7254 ) ;
#13343=CARTESIAN_POINT ( 'NONE',  ( -70.92837670882107659, -27.85319909218681644, -6.138794830819693793 ) ) ;
#13376=VECTOR ( 'NONE', #28065, 1000.000000000000000 ) ;
#13379=EDGE_LOOP ( 'NONE', ( #11149, #13464 ) ) ;
#13394=ADVANCED_FACE ( 'NONE', ( #4915 ), #17446, .T. ) ;
#13442=CARTESIAN_POINT ( 'NONE',  ( -70.92837670882107659, 28.72470171467712063, -4.357836081054403010 ) ) ;
#13464=ORIENTED_EDGE ( 'NONE', *, *, #21751, .T. ) ;
#13488=EDGE_CURVE ( 'NONE', #39731, #10043, #12721, .T. ) ;
#13536=VECTOR ( 'NONE', #3782, 1000.000000000000000 ) ;
#13611=CARTESIAN_POINT ( 'NONE',  ( -70.66586135525236045, 0.1905911290138092018, 5.995467141624639673 ) ) ;
#13707=ORIENTED_EDGE ( 'NONE', *, *, #20042, .F. ) ;
#13708=CARTESIAN_POINT ( 'NONE',  ( -70.92837670882107659, 26.72470171467712063, 6.406751979251626317 ) ) ;
#13752=ORIENTED_EDGE ( 'NONE', *, *, #3898, .T. ) ;
#13755=ORIENTED_EDGE ( 'NONE', *, *, #26456, .T. ) ;
#13772=VECTOR ( 'NONE', #84, 1000.000000000000114 ) ;
#13788=CARTESIAN_POINT ( 'NONE',  ( -70.92837670882107659, -27.85319909218681644, -4.357836081054403010 ) ) ;
#13804=( NAMED_UNIT ( * ) PLANE_ANGLE_UNIT ( ) SI_UNIT ( $, .RADIAN. ) );
#13852=EDGE_CURVE ( 'NONE', #27757, #30983, #11533, .T. ) ;
#13945=ADVANCED_FACE ( 'NONE', ( #28115 ), #18635, .T. ) ;
#14039=EDGE_CURVE ( 'NONE', #462, #5317, #15497, .T. ) ;
#14046=CARTESIAN_POINT ( 'NONE',  ( -70.92837670882107659, 28.72470171467712063, -2.000000000000000000 ) ) ;
#14127=AXIS2_PLACEMENT_3D ( 'NONE', #23261, #10285, #3739 ) ;
#14141=CARTESIAN_POINT ( 'NONE',  ( -71.64402667994158946, -21.49031309831630665, 3.957576123060442708 ) ) ;
#14181=DIRECTION ( 'NONE',  ( -0.000000000000000000, 1.000000000000000000, -0.000000000000000000 ) ) ;
#14235=CARTESIAN_POINT ( 'NONE',  ( -70.81198565705318515, 0.2164538760997103128, 6.011900603202949611 ) ) ;
#14369=AXIS2_PLACEMENT_3D ( 'NONE', #36666, #8448, #21646 ) ;
#14373=DIRECTION ( 'NONE',  ( -0.000000000000000000, 1.000000000000000000, -0.000000000000000000 ) ) ;
#14380=VERTEX_POINT ( 'NONE', #19305 ) ;
#14393=ORIENTED_EDGE ( 'NONE', *, *, #33110, .F. ) ;
#14433=CARTESIAN_POINT ( 'NONE',  ( -70.02024225408199243, -0.3498828673826461233, 3.930990725878107384 ) ) ;
#14440=CONICAL_SURFACE ( 'NONE', #36174, 6.406751979251626317, 0.7853981633974482790 ) ;
#14463=CARTESIAN_POINT ( 'NONE',  ( -70.92837670882107659, 26.72470171467712063, 0.000000000000000000 ) ) ;
#14525=DIRECTION ( 'NONE',  ( -0.000000000000000000, 1.000000000000000000, -0.000000000000000000 ) ) ;
#14536=CARTESIAN_POINT ( 'NONE',  ( -71.92837670882107659, -20.78299143688747819, 3.916079783099609912 ) ) ;
#14542=DIRECTION ( 'NONE',  ( 0.000000000000000000, 0.000000000000000000, 1.000000000000000000 ) ) ;
#14553=ORIENTED_EDGE ( 'NONE', *, *, #35846, .T. ) ;
#14609=CARTESIAN_POINT ( 'NONE',  ( -70.92837670882107659, 28.72470171467712063, 6.000000000000005329 ) ) ;
#14625=DIRECTION ( 'NONE',  ( -0.000000000000000000, 1.000000000000000000, -0.000000000000000000 ) ) ;
#14628=CARTESIAN_POINT ( 'NONE',  ( -70.29787437547823004, 0.001187990818876110462, 5.979574859000733156 ) ) ;
#14672=CARTESIAN_POINT ( 'NONE',  ( -71.54330396476282772, 0.01623308404284228706, 3.969121680875197455 ) ) ;
#14721=CARTESIAN_POINT ( 'NONE',  ( -70.05472099546194897, -0.2795093347480433477, 3.936269516561393456 ) ) ;
#14793=ORIENTED_EDGE ( 'NONE', *, *, #13852, .T. ) ;
#14799=EDGE_CURVE ( 'NONE', #8440, #34705, #21332, .T. ) ;
#14837=CARTESIAN_POINT ( 'NONE',  ( -71.45635794260526552, 0.07346082103169225552, 3.977567636976454768 ) ) ;
#14850=ORIENTED_EDGE ( 'NONE', *, *, #8540, .F. ) ;
#14957=CARTESIAN_POINT ( 'NONE',  ( -70.60020594839741648, -21.73402473355089271, 3.991851897078962708 ) ) ;
#14976=DIRECTION ( 'NONE',  ( -0.000000000000000000, 0.000000000000000000, 1.000000000000000000 ) ) ;
#15088=CARTESIAN_POINT ( 'NONE',  ( -71.72837670882105954, -34.30579396504363388, -1.385640646055078307 ) ) ;
#15161=CARTESIAN_POINT ( 'NONE',  ( -71.15343164110390717, -21.75733751372833069, 3.995777704139396036 ) ) ;
#15167=ORIENTED_EDGE ( 'NONE', *, *, #35067, .T. ) ;
#15168=AXIS2_PLACEMENT_3D ( 'NONE', #23162, #1962, #10983 ) ;
#15181=CARTESIAN_POINT ( 'NONE',  ( -70.92837670882107659, 15.04836564048558500, 0.000000000000000000 ) ) ;
#15191=EDGE_CURVE ( 'NONE', #25957, #7083, #18582, .T. ) ;
#15255=CARTESIAN_POINT ( 'NONE',  ( -71.45635794260526552, 0.07346082103169225552, 5.989611775372480018 ) ) ;
#15341=DIRECTION ( 'NONE',  ( 0.000000000000000000, 0.000000000000000000, 1.000000000000000000 ) ) ;
#15365=CARTESIAN_POINT ( 'NONE',  ( -70.30712919725708332, -21.57437711518543111, 3.968280824155048236 ) ) ;
#15455=CARTESIAN_POINT ( 'NONE',  ( -71.77605803285275954, -0.2407680685837292611, 3.940028962036595139 ) ) ;
#15497=CIRCLE ( 'NONE', #25350, 6.000000000000005329 ) ;
#15515=ORIENTED_EDGE ( 'NONE', *, *, #22898, .T. ) ;
#15547=FACE_BOUND ( 'NONE', #40416, .T. ) ;
#15561=CONICAL_SURFACE ( 'NONE', #20809, 6.138794830819693793, 0.03429555972217021576 ) ;
#15566=AXIS2_PLACEMENT_3D ( 'NONE', #7842, #19995, #10715 ) ;
#15591=( GEOMETRIC_REPRESENTATION_CONTEXT ( 3 ) GLOBAL_UNCERTAINTY_ASSIGNED_CONTEXT ( ( #24225 ) ) GLOBAL_UNIT_ASSIGNED_CONTEXT ( ( #4937, #13804, #10499 ) ) REPRESENTATION_CONTEXT ( 'NONE', 'WORKASPACE' ) );
#15612=CARTESIAN_POINT ( 'NONE',  ( -71.92837670882107659, -0.7829914368874774100, 5.916079783099621459 ) ) ;
#15744=B_SPLINE_CURVE_WITH_KNOTS ( 'NONE', 3,
 ( #24959, #37493, #38109, #34655, #6427, #16090, #22492, #16287, #31546, #19182 ),
 .UNSPECIFIED., .F., .F.,
 ( 4, 2, 2, 2, 4 ),
 ( 0.5001220714135948819, 0.6250915535601961892, 0.7500610357067973855, 0.8750305178533986927, 1.000000000000000000 ),
 .UNSPECIFIED. ) ;
#15811=EDGE_LOOP ( 'NONE', ( #20782, #13707, #33619 ) ) ;
#15814=ORIENTED_EDGE ( 'NONE', *, *, #11832, .T. ) ;
#15818=FACE_OUTER_BOUND ( 'NONE', #37796, .T. ) ;
#15839=VECTOR ( 'NONE', #17409, 1000.000000000000000 ) ;
#15942=DIRECTION ( 'NONE',  ( -0.000000000000000000, 1.000000000000000000, -0.000000000000000000 ) ) ;
#16025=VERTEX_POINT ( 'NONE', #15612 ) ;
#16090=CARTESIAN_POINT ( 'NONE',  ( -70.12981335532620619, -21.39869996748758396, 3.947339383427191262 ) ) ;
#16158=AXIS2_PLACEMENT_3D ( 'NONE', #12676, #9180, #22173 ) ;
#16167=CARTESIAN_POINT ( 'NONE',  ( -70.92837670882107659, 26.72470171467712063, -6.406751979251626317 ) ) ;
#16287=CARTESIAN_POINT ( 'NONE',  ( -69.95498688392430608, -21.04617888798872727, 3.920732911918689556 ) ) ;
#16289=VERTEX_POINT ( 'NONE', #21911 ) ;
#16291=CARTESIAN_POINT ( 'NONE',  ( -70.92837670882107659, 15.04836564048558500, -6.406751979251626317 ) ) ;
#16316=CARTESIAN_POINT ( 'NONE',  ( -69.92837670882107659, 28.72470171467712063, 5.916079783099620570 ) ) ;
#16412=AXIS2_PLACEMENT_3D ( 'NONE', #30913, #20324, #23625 ) ;
#16619=ORIENTED_EDGE ( 'NONE', *, *, #76, .F. ) ;
#16722=DIRECTION ( 'NONE',  ( -0.000000000000000000, 1.000000000000000000, -0.000000000000000000 ) ) ;
#16771=CARTESIAN_POINT ( 'NONE',  ( -70.92837670882107659, 15.04836564048558500, 0.000000000000000000 ) ) ;
#16776=VECTOR ( 'NONE', #10453, 1000.000000000000114 ) ;
#16834=CARTESIAN_POINT ( 'NONE',  ( -70.92837670882107659, 15.04836564048558500, 6.406751979251626317 ) ) ;
#16886=CARTESIAN_POINT ( 'NONE',  ( -70.42518435975088664, 0.09082038125507381487, 5.980078429000515783 ) ) ;
#16944=CARTESIAN_POINT ( 'NONE',  ( -71.72837670882105954, -34.30579396504363388, 1.385640646055090519 ) ) ;
#17000=FACE_OUTER_BOUND ( 'NONE', #5988, .T. ) ;
#17007=DIRECTION ( 'NONE',  ( 0.000000000000000000, -1.000000000000000000, 0.000000000000000000 ) ) ;
#17065=DIRECTION ( 'NONE',  ( 0.000000000000000000, -1.000000000000000000, 0.000000000000000000 ) ) ;
#17126=ORIENTED_EDGE ( 'NONE', *, *, #10815, .F. ) ;
#17179=EDGE_CURVE ( 'NONE', #39825, #38785, #810, .T. ) ;
#17202=CARTESIAN_POINT ( 'NONE',  ( -70.92837670882107659, 28.72470171467712063, 0.000000000000000000 ) ) ;
#17249=CARTESIAN_POINT ( 'NONE',  ( -70.92837670882107659, 13.87661300689593880, 0.000000000000000000 ) ) ;
#17307=CARTESIAN_POINT ( 'NONE',  ( -71.72837670882105954, -34.30579396504363388, -1.385640646055078307 ) ) ;
#17310=CARTESIAN_POINT ( 'NONE',  ( -70.70332177653823180, 0.1913546399533780362, 6.007821842535422618 ) ) ;
#17316=DIRECTION ( 'NONE',  ( -0.000000000000000000, 1.000000000000000000, -0.000000000000000000 ) ) ;
#17320=DIRECTION ( 'NONE',  ( -0.8660254037844381525, 0.000000000000000000, 0.5000000000000008882 ) ) ;
#17334=VECTOR ( 'NONE', #6822, 1000.000000000000000 ) ;
#17409=DIRECTION ( 'NONE',  ( -0.000000000000000000, 1.000000000000000000, -0.000000000000000000 ) ) ;
#17415=FACE_OUTER_BOUND ( 'NONE', #37883, .T. ) ;
#17438=DIRECTION ( 'NONE',  ( -0.4999999999999986122, 0.000000000000000000, 0.8660254037844394848 ) ) ;
#17446=CYLINDRICAL_SURFACE ( 'NONE', #2318, 3.784187430299790211 ) ;
#17509=CARTESIAN_POINT ( 'NONE',  ( -69.92837670882107659, -0.7829914368874777431, 5.928123921495636495 ) ) ;
#17602=ADVANCED_BREP_SHAPE_REPRESENTATION ( '', ( #12327, #30744 ), #15591 ) ;
#17623=CARTESIAN_POINT ( 'NONE',  ( -71.83651116356016075, -21.21610000639230975, 5.943034864274126861 ) ) ;
#17716=DIRECTION ( 'NONE',  ( -0.000000000000000000, 1.000000000000000000, -0.000000000000000000 ) ) ;
#17828=CARTESIAN_POINT ( 'NONE',  ( -70.40039547503687345, -21.63944369480664776, 5.989611775372475577 ) ) ;
#17839=CARTESIAN_POINT ( 'NONE',  ( -70.79777098150788106, -21.78301052427940832, 6.000000000000010658 ) ) ;
#17905=LINE ( 'NONE', #14609, #8310 ) ;
#17925=CARTESIAN_POINT ( 'NONE',  ( -71.54962422038506986, 0.008394241410477492477, 3.968280824155049125 ) ) ;
#18009=FACE_OUTER_BOUND ( 'NONE', #1615, .T. ) ;
#18021=CARTESIAN_POINT ( 'NONE',  ( -70.66492681425577871, 0.2167243893765767038, 4.000000000152813762 ) ) ;
#18051=CARTESIAN_POINT ( 'NONE',  ( -71.92837670882107659, 28.72470171467712063, 5.916079783099620570 ) ) ;
#18130=CARTESIAN_POINT ( 'NONE',  ( -71.70854571598145810, -0.1474806467180565794, 3.949606264851800663 ) ) ;
#18139=CARTESIAN_POINT ( 'NONE',  ( -70.92837670882140344, -21.78291075931342391, 6.000000000000002665 ) ) ;
#18163=VECTOR ( 'NONE', #11198, 1000.000000000000114 ) ;
#18177=CARTESIAN_POINT ( 'NONE',  ( -67.14418927852128149, 15.04836564048558500, 0.000000000000000000 ) ) ;
#18243=CARTESIAN_POINT ( 'NONE',  ( -70.08069538478937943, -21.32521480519122647, 5.952073100432614616 ) ) ;
#18245=ORIENTED_EDGE ( 'NONE', *, *, #15191, .T. ) ;
#18332=CARTESIAN_POINT ( 'NONE',  ( -70.92661119047551210, 0.2232129446074198609, 4.001025162589364470 ) ) ;
#18343=B_SPLINE_SURFACE_WITH_KNOTS ( 'NONE', 3, 1, ( 
 ( #17509, #29497 ),
 ( #4395, #30103 ),
 ( #26606, #11334 ),
 ( #26807, #23315 ),
 ( #24107, #14433 ),
 ( #27004, #39550 ),
 ( #4775, #30298 ),
 ( #11137, #2112 ),
 ( #14628, #32598 ),
 ( #1306, #23708 ),
 ( #26412, #39143 ),
 ( #38941, #23518 ),
 ( #17310, #1704 ),
 ( #14235, #27609 ),
 ( #3150, #18332 ),
 ( #40166, #36671 ),
 ( #34428, #11947 ),
 ( #8454, #21038 ),
 ( #11737, #27807 ),
 ( #15255, #14837 ),
 ( #31124, #17925 ),
 ( #9274, #8659 ),
 ( #2314, #18130 ),
 ( #21651, #15455 ),
 ( #30508, #9075 ),
 ( #39967, #21852 ),
 ( #40563, #33611 ),
 ( #21236, #37283 ),
 ( #30924, #5385 ),
 ( #27404, #2731 ),
 ( #36879, #24315 ) ),
 .UNSPECIFIED., .F., .F., .F.,
 ( 4, 3, 3, 3, 3, 3, 3, 3, 3, 3, 4 ),
 ( 2, 2 ),
 ( 0.000000000000000000, 0.1064040534484947675, 0.2127447817800691698, 0.3200334471358571298, 0.4279895727010789019, 0.5349334657245100599, 0.6407861787064421666, 0.7471238984184978005, 0.8547834834472670673, 0.9625789755878069176, 1.000000000000000000 ),
 ( 0.000000000000000000, 1.000000000000000000 ),
 .UNSPECIFIED. ) ;
#18389=CARTESIAN_POINT ( 'NONE',  ( -70.92837670882140344, -21.78291075931342391, 6.000000000000002665 ) ) ;
#18420=DIRECTION ( 'NONE',  ( 0.000000000000000000, 0.000000000000000000, 1.000000000000000000 ) ) ;
#18505=CARTESIAN_POINT ( 'NONE',  ( -70.92837670882107659, 26.72470171467712063, 0.000000000000000000 ) ) ;
#18564=DIRECTION ( 'NONE',  ( 0.000000000000000000, -1.000000000000000000, 0.000000000000000000 ) ) ;
#18582=LINE ( 'NONE', #40011, #13376 ) ;
#18635=CYLINDRICAL_SURFACE ( 'NONE', #22100, 6.000000000000005329 ) ;
#18647=ORIENTED_EDGE ( 'NONE', *, *, #14039, .F. ) ;
#18651=CARTESIAN_POINT ( 'NONE',  ( -69.93541594206888590, -20.90143516061696616, 5.929309462487109883 ) ) ;
#18698=APPLICATION_CONTEXT ( 'automotive_design' ) ;
#18708=CARTESIAN_POINT ( 'NONE',  ( -71.19001092293638067, 0.1909006763965998277, 5.995522264747400243 ) ) ;
#18724=EDGE_CURVE ( 'NONE', #36751, #16025, #25367, .T. ) ;
#18736=CIRCLE ( 'NONE', #31897, 6.406751979251626317 ) ;
#18849=CARTESIAN_POINT ( 'NONE',  ( -70.92837670882107659, -27.85319909218681644, 6.138794830819693793 ) ) ;
#18858=AXIS2_PLACEMENT_3D ( 'NONE', #28372, #32096, #12720 ) ;
#18932=VECTOR ( 'NONE', #9818, 1000.000000000000000 ) ;
#18944=ORIENTED_EDGE ( 'NONE', *, *, #28941, .T. ) ;
#18977=CYLINDRICAL_SURFACE ( 'NONE', #20581, 6.406751979251626317 ) ;
#19057=DIRECTION ( 'NONE',  ( -0.000000000000000000, 1.000000000000000000, -0.000000000000000000 ) ) ;
#19068=CYLINDRICAL_SURFACE ( 'NONE', #16158, 4.357836081054403010 ) ;
#19165=ORIENTED_EDGE ( 'NONE', *, *, #26456, .F. ) ;
#19182=CARTESIAN_POINT ( 'NONE',  ( -69.92837670882107659, -20.78299143688747819, 3.916079783099623679 ) ) ;
#19217=FACE_OUTER_BOUND ( 'NONE', #19924, .T. ) ;
#19271=FACE_OUTER_BOUND ( 'NONE', #32466, .T. ) ;
#19277=DIRECTION ( 'NONE',  ( -0.000000000000000000, 1.000000000000000000, -0.000000000000000000 ) ) ;
#19305=CARTESIAN_POINT ( 'NONE',  ( -69.32837670882108227, -34.30579396504363388, 1.870248747537495149E-15 ) ) ;
#19383=ORIENTED_EDGE ( 'NONE', *, *, #8570, .F. ) ;
#19395=ORIENTED_EDGE ( 'NONE', *, *, #17179, .F. ) ;
#19536=CARTESIAN_POINT ( 'NONE',  ( -71.43233049654038780, 0.09072970090432713741, 5.980030958859732237 ) ) ;
#19600=CARTESIAN_POINT ( 'NONE',  ( -70.79764455194573713, 0.2168280239975503842, 5.999999999999999112 ) ) ;
#19620=CARTESIAN_POINT ( 'NONE',  ( -69.32837670882108227, -34.30579396504363388, 1.870248747537495149E-15 ) ) ;
#19794=CARTESIAN_POINT ( 'NONE',  ( -69.95447152169636240, -0.5205953579843026757, 5.920650877785231359 ) ) ;
#19819=CARTESIAN_POINT ( 'NONE',  ( -70.92837670882107659, 15.04836564048558500, 3.784187430299790211 ) ) ;
#19924=EDGE_LOOP ( 'NONE', ( #14850, #15167, #36617, #306, #22089, #23531, #15814, #10888 ) ) ;
#19995=DIRECTION ( 'NONE',  ( 0.000000000000000000, -1.000000000000000000, 0.000000000000000000 ) ) ;
#20042=EDGE_CURVE ( 'NONE', #33142, #3556, #25425, .T. ) ;
#20184=DIRECTION ( 'NONE',  ( -0.000000000000000000, 1.000000000000000000, -0.000000000000000000 ) ) ;
#20268=CIRCLE ( 'NONE', #2557, 3.784187430299790211 ) ;
#20284=ORIENTED_EDGE ( 'NONE', *, *, #40617, .F. ) ;
#20300=DIRECTION ( 'NONE',  ( 0.000000000000000000, -0.000000000000000000, -1.000000000000000000 ) ) ;
#20324=DIRECTION ( 'NONE',  ( -0.000000000000000000, 1.000000000000000000, -0.000000000000000000 ) ) ;
#20378=AXIS2_PLACEMENT_3D ( 'NONE', #34250, #6023, #34044 ) ;
#20405=CARTESIAN_POINT ( 'NONE',  ( -70.92837670882107659, 28.72470171467712063, 0.000000000000000000 ) ) ;
#20406=FACE_OUTER_BOUND ( 'NONE', #8259, .T. ) ;
#20520=VECTOR ( 'NONE', #22725, 1000.000000000000000 ) ;
#20526=CARTESIAN_POINT ( 'NONE',  ( -69.32837670882108227, -31.30579396504363388, 1.870248747537495149E-15 ) ) ;
#20533=ADVANCED_FACE ( 'NONE', ( #30232 ), #11069, .F. ) ;
#20543=DIRECTION ( 'NONE',  ( -0.000000000000000000, 1.000000000000000000, -0.000000000000000000 ) ) ;
#20581=AXIS2_PLACEMENT_3D ( 'NONE', #28438, #2950, #28027 ) ;
#20782=ORIENTED_EDGE ( 'NONE', *, *, #11043, .F. ) ;
#20809=AXIS2_PLACEMENT_3D ( 'NONE', #853, #17065, #25961 ) ;
#20901=FACE_OUTER_BOUND ( 'NONE', #32313, .T. ) ;
#20933=VECTOR ( 'NONE', #1788, 1000.000000000000114 ) ;
#20941=CARTESIAN_POINT ( 'NONE',  ( -70.92837670882107659, 15.04836564048558500, 0.000000000000000000 ) ) ;
#21005=CARTESIAN_POINT ( 'NONE',  ( -70.92837670882107659, 13.87661300689593880, -6.000000000000005329 ) ) ;
#21020=CARTESIAN_POINT ( 'NONE',  ( -70.92837670882107659, 13.87661300689593880, 0.000000000000000000 ) ) ;
#21027=ADVANCED_FACE ( 'NONE', ( #17000 ), #33285, .T. ) ;
#21038=CARTESIAN_POINT ( 'NONE',  ( -71.25654746924473670, 0.1680418597759353594, 3.991851897078962708 ) ) ;
#21139=DIRECTION ( 'NONE',  ( 0.000000000000000000, 0.000000000000000000, 1.000000000000000000 ) ) ;
#21147=CARTESIAN_POINT ( 'NONE',  ( -70.08069538478937943, -21.32521480519122647, 3.940028962036594251 ) ) ;
#21163=DIRECTION ( 'NONE',  ( -1.000000000000000000, 0.000000000000000000, -0.000000000000000000 ) ) ;
#21233=DIRECTION ( 'NONE',  ( 0.000000000000000000, 0.000000000000000000, 1.000000000000000000 ) ) ;
#21236=CARTESIAN_POINT ( 'NONE',  ( -71.92133747557326728, -0.6645477131579885510, 5.929309462487116100 ) ) ;
#21245=CARTESIAN_POINT ( 'NONE',  ( -71.43156905789128075, -21.65680325503002734, 5.980078429000514006 ) ) ;
#21264=ORIENTED_EDGE ( 'NONE', *, *, #9302, .F. ) ;
#21271=ORIENTED_EDGE ( 'NONE', *, *, #23474, .T. ) ;
#21289=PLANE ( 'NONE',  #24803 ) ;
#21332=LINE ( 'NONE', #25239, #33108 ) ;
#21351=CARTESIAN_POINT ( 'NONE',  ( -69.92837670882107659, -20.78299143688747819, 3.916079783099620126 ) ) ;
#21564=ORIENTED_EDGE ( 'NONE', *, *, #18724, .T. ) ;
#21565=CARTESIAN_POINT ( 'NONE',  ( -70.22814611767556414, -21.49690818219047017, 5.971043812772915516 ) ) ;
#21646=DIRECTION ( 'NONE',  ( 0.000000000000000000, -0.000000000000000000, -1.000000000000000000 ) ) ;
#21651=CARTESIAN_POINT ( 'NONE',  ( -71.77605803285275954, -0.2407680685837292611, 5.952073100432620834 ) ) ;
#21660=CARTESIAN_POINT ( 'NONE',  ( -71.19089206238980694, -21.75657400278875286, 5.995467141624637009 ) ) ;
#21667=AXIS2_PLACEMENT_3D ( 'NONE', #473, #18564, #21681 ) ;
#21681=DIRECTION ( 'NONE',  ( 0.000000000000000000, 0.000000000000000000, -1.000000000000000000 ) ) ;
#21705=VECTOR ( 'NONE', #27505, 1000.000000000000114 ) ;
#21730=ORIENTED_EDGE ( 'NONE', *, *, #10815, .T. ) ;
#21751=EDGE_CURVE ( 'NONE', #8622, #1010, #7509, .T. ) ;
#21762=CARTESIAN_POINT ( 'NONE',  ( -70.50053432363721129, -21.68684479525939324, 3.984726467720987042 ) ) ;
#21778=LINE ( 'NONE', #34357, #18932 ) ;
#21791=EDGE_LOOP ( 'NONE', ( #34050, #25510 ) ) ;
#21852=CARTESIAN_POINT ( 'NONE',  ( -71.87513448197603338, -0.4420453205300980959, 3.925045345733726432 ) ) ;
#21911=CARTESIAN_POINT ( 'NONE',  ( -70.92837670224925262, -21.78291075600659354, 3.999987187540717137 ) ) ;
#21965=PRODUCT_DEFINITION ( 'UNKNOWN', '', #35365, #31238 ) ;
#22089=ORIENTED_EDGE ( 'NONE', *, *, #4058, .T. ) ;
#22100=AXIS2_PLACEMENT_3D ( 'NONE', #8958, #25041, #37775 ) ;
#22142=DIRECTION ( 'NONE',  ( -0.000000000000000000, 1.000000000000000000, -0.000000000000000000 ) ) ;
#22173=DIRECTION ( 'NONE',  ( 0.000000000000000000, 0.000000000000000000, 1.000000000000000000 ) ) ;
#22254=EDGE_CURVE ( 'NONE', #25957, #9702, #9697, .T. ) ;
#22479=LINE ( 'NONE', #28644, #17334 ) ;
#22492=CARTESIAN_POINT ( 'NONE',  ( -70.05509079466530409, -21.28757458321500451, 3.936323582624761119 ) ) ;
#22537=EDGE_LOOP ( 'NONE', ( #4138, #17126 ) ) ;
#22660=ORIENTED_EDGE ( 'NONE', *, *, #125, .T. ) ;
#22684=ORIENTED_EDGE ( 'NONE', *, *, #4058, .F. ) ;
#22696=FACE_OUTER_BOUND ( 'NONE', #27665, .T. ) ;
#22725=DIRECTION ( 'NONE',  ( -0.000000000000000000, 1.000000000000000000, -0.000000000000000000 ) ) ;
#22731=LINE ( 'NONE', #35295, #37709 ) ;
#22756=ORIENTED_EDGE ( 'NONE', *, *, #6630, .F. ) ;
#22880=ORIENTED_EDGE ( 'NONE', *, *, #13488, .F. ) ;
#22898=EDGE_CURVE ( 'NONE', #23332, #5710, #18736, .T. ) ;
#22912=PLANE ( 'NONE',  #30267 ) ;
#22948=CARTESIAN_POINT ( 'NONE',  ( -69.92837670882107659, -0.7829914368874778541, 3.916079783099621014 ) ) ;
#23065=DIRECTION ( 'NONE',  ( 0.000000000000000000, 0.000000000000000000, 1.000000000000000000 ) ) ;
#23162=CARTESIAN_POINT ( 'NONE',  ( -71.72837670882105954, -34.30579396504363388, 1.385640646055090519 ) ) ;
#23261=CARTESIAN_POINT ( 'NONE',  ( -70.92837670882107659, 28.72470171467712063, 0.000000000000000000 ) ) ;
#23263=FACE_OUTER_BOUND ( 'NONE', #11721, .T. ) ;
#23315=CARTESIAN_POINT ( 'NONE',  ( -69.98383490720681266, -0.4546002296310912572, 3.925186983125784401 ) ) ;
#23332=VERTEX_POINT ( 'NONE', #16291 ) ;
#23335=CARTESIAN_POINT ( 'NONE',  ( -70.92837670882107659, 13.87661300689593880, -3.784187430299790211 ) ) ;
#23354=( LENGTH_UNIT ( ) NAMED_UNIT ( * ) SI_UNIT ( .MILLI., .METRE. ) );
#23468=FACE_OUTER_BOUND ( 'NONE', #30911, .T. ) ;
#23474=EDGE_CURVE ( 'NONE', #5710, #23332, #955, .T. ) ;
#23518=CARTESIAN_POINT ( 'NONE',  ( -70.59363788503038961, 0.1660198011701667642, 3.991660656778088789 ) ) ;
#23531=ORIENTED_EDGE ( 'NONE', *, *, #18724, .F. ) ;
#23605=CARTESIAN_POINT ( 'NONE',  ( -70.92837670882107659, 26.72470171467712063, 0.000000000000000000 ) ) ;
#23625=DIRECTION ( 'NONE',  ( 0.000000000000000000, 0.000000000000000000, 1.000000000000000000 ) ) ;
#23676=LINE ( 'NONE', #7423, #10114 ) ;
#23688=PLANE ( 'NONE',  #15566 ) ;
#23708=CARTESIAN_POINT ( 'NONE',  ( -70.39213229241123315, 0.06107131307206801335, 3.975988782274378686 ) ) ;
#23720=DIRECTION ( 'NONE',  ( 0.000000000000000000, 0.000000000000000000, 1.000000000000000000 ) ) ;
#23815=CARTESIAN_POINT ( 'NONE',  ( -69.92837670882107659, -20.78299143688747819, 5.916079783099621459 ) ) ;
#23841=VERTEX_POINT ( 'NONE', #20526 ) ;
#23934=DIRECTION ( 'NONE',  ( 0.000000000000000000, 0.000000000000000000, 1.000000000000000000 ) ) ;
#23959=CARTESIAN_POINT ( 'NONE',  ( -71.92837670882107659, 28.72470171467712063, 3.916079783099620126 ) ) ;
#23987=DIRECTION ( 'NONE',  ( 0.000000000000000000, 0.000000000000000000, 1.000000000000000000 ) ) ;
#24008=CARTESIAN_POINT ( 'NONE',  ( -69.93073207689441517, -20.86216845902604078, 5.928523475362944772 ) ) ;
#24068=ORIENTED_EDGE ( 'NONE', *, *, #5170, .T. ) ;
#24102=CONICAL_SURFACE ( 'NONE', #18858, 6.138794830819693793, 0.03429555972217021576 ) ;
#24104=CARTESIAN_POINT ( 'NONE',  ( -69.92837670882107659, -0.7829914368874778541, 5.916079783099621459 ) ) ;
#24107=CARTESIAN_POINT ( 'NONE',  ( -70.02024225408199243, -0.3498828673826461233, 5.943034864274133078 ) ) ;
#24208=DIRECTION ( 'NONE',  ( 0.000000000000000000, 0.000000000000000000, 1.000000000000000000 ) ) ;
#24224=CARTESIAN_POINT ( 'NONE',  ( -70.22814611767556414, -21.49690818219047017, 3.958999674376895150 ) ) ;
#24225=UNCERTAINTY_MEASURE_WITH_UNIT (LENGTH_MEASURE( 1.000000000000000082E-05 ), #4937, 'distance_accuracy_value', 'NONE');
#24238=PLANE ( 'NONE',  #3809 ) ;
#24268=DIRECTION ( 'NONE',  ( 0.000000000000000000, 0.000000000000000000, 1.000000000000000000 ) ) ;
#24286=CARTESIAN_POINT ( 'NONE',  ( -70.92837670224925262, -21.78291075600659354, 3.999987187540717137 ) ) ;
#24315=CARTESIAN_POINT ( 'NONE',  ( -71.92837670882107659, -0.7829914368874768549, 3.916079783099621014 ) ) ;
#24380=B_SPLINE_SURFACE_WITH_KNOTS ( 'NONE', 3, 1, ( 
 ( #1607, #14536 ),
 ( #36382, #39250 ),
 ( #32701, #4501 ),
 ( #29599, #35987 ),
 ( #17623, #5088 ),
 ( #1414, #7769 ),
 ( #30199, #32901 ),
 ( #4688, #14141 ),
 ( #27110, #11042 ),
 ( #1814, #39660 ),
 ( #11442, #35597 ),
 ( #7367, #3059 ),
 ( #2844, #15161 ),
 ( #30409, #11647 ),
 ( #33714, #11856 ),
 ( #6116, #37394 ),
 ( #8568, #24432 ),
 ( #9188, #14957 ),
 ( #31038, #21762 ),
 ( #17828, #40272 ),
 ( #2436, #15365 ),
 ( #21565, #24224 ),
 ( #27921, #8978 ),
 ( #18243, #21147 ),
 ( #5493, #40684 ),
 ( #24635, #36784 ),
 ( #40077, #36986 ),
 ( #18651, #8768 ),
 ( #24008, #36583 ),
 ( #5703, #27525 ),
 ( #2218, #21351 ) ),
 .UNSPECIFIED., .F., .F., .F.,
 ( 4, 3, 3, 3, 3, 3, 3, 3, 3, 3, 4 ),
 ( 2, 2 ),
 ( 0.000000000000000000, 0.1064040534484947120, 0.2127447817800686702, 0.3200334471358569077, 0.4279895727010785689, 0.5349334657245098379, 0.6407861787064418335, 0.7471238984184976895, 0.8547834834472671783, 0.9625789755878066956, 1.000000000000000000 ),
 ( 0.000000000000000000, 1.000000000000000000 ),
 .UNSPECIFIED. ) ;
#24414=CARTESIAN_POINT ( 'NONE',  ( -70.12865035339947894, -0.1685304919200742435, 3.947195235540182701 ) ) ;
#24432=CARTESIAN_POINT ( 'NONE',  ( -70.70940173728274658, -21.76495738335424690, 3.997008894667204881 ) ) ;
#24444=EDGE_CURVE ( 'NONE', #38572, #10250, #22731, .T. ) ;
#24520=CARTESIAN_POINT ( 'NONE',  ( -70.92837670882107659, 13.87661300689593880, 0.000000000000000000 ) ) ;
#24521=ORIENTED_EDGE ( 'NONE', *, *, #6142, .T. ) ;
#24635=CARTESIAN_POINT ( 'NONE',  ( -69.98161893566610559, -21.12393755324485412, 5.937089484129746353 ) ) ;
#24638=AXIS2_PLACEMENT_3D ( 'NONE', #17202, #10823, #5066 ) ;
#24678=ORIENTED_EDGE ( 'NONE', *, *, #76, .T. ) ;
#24789=EDGE_CURVE ( 'NONE', #10043, #3556, #22479, .T. ) ;
#24803=AXIS2_PLACEMENT_3D ( 'NONE', #4483, #17007, #20300 ) ;
#24959=CARTESIAN_POINT ( 'NONE',  ( -70.92837670224925262, -21.78291075600659354, 3.999987187540717137 ) ) ;
#25041=DIRECTION ( 'NONE',  ( -0.000000000000000000, 1.000000000000000000, -0.000000000000000000 ) ) ;
#25063=ORIENTED_EDGE ( 'NONE', *, *, #11054, .F. ) ;
#25239=CARTESIAN_POINT ( 'NONE',  ( -70.92837670882107659, 28.72470171467712063, 3.784187430299790211 ) ) ;
#25350=AXIS2_PLACEMENT_3D ( 'NONE', #17249, #20543, #8390 ) ;
#25365=ORIENTED_EDGE ( 'NONE', *, *, #24789, .F. ) ;
#25367=B_SPLINE_CURVE_WITH_KNOTS ( 'NONE', 3,
 ( #28600, #25512, #18708, #19536, #35204, #38058, #12737, #611, #37636, #25713 ),
 .UNSPECIFIED., .F., .F.,
 ( 4, 2, 2, 2, 4 ),
 ( 0.001566344281586673362, 0.001957551653609702468, 0.002348759025632731357, 0.002739966397655760246, 0.003131173769678789135 ),
 .UNSPECIFIED. ) ;
#25378=CARTESIAN_POINT ( 'NONE',  ( -70.92837670882107659, 15.04836564048558500, -3.784187430299790211 ) ) ;
#25401=CARTESIAN_POINT ( 'NONE',  ( -70.92837670882107659, 28.72470171467712063, 6.406751979251626317 ) ) ;
#25425=LINE ( 'NONE', #38170, #32533 ) ;
#25510=ORIENTED_EDGE ( 'NONE', *, *, #7116, .T. ) ;
#25512=CARTESIAN_POINT ( 'NONE',  ( -71.05898243613420107, 0.2170276505044492765, 6.000000000000012434 ) ) ;
#25526=ORIENTED_EDGE ( 'NONE', *, *, #8074, .F. ) ;
#25648=VECTOR ( 'NONE', #11000, 1000.000000000000000 ) ;
#25666=ORIENTED_EDGE ( 'NONE', *, *, #35615, .F. ) ;
#25713=CARTESIAN_POINT ( 'NONE',  ( -71.92837670882107659, -0.7829914368874774100, 5.916079783099621459 ) ) ;
#25812=EDGE_CURVE ( 'NONE', #14380, #39731, #36486, .T. ) ;
#25840=( NAMED_UNIT ( * ) PLANE_ANGLE_UNIT ( ) SI_UNIT ( $, .RADIAN. ) );
#25939=ORIENTED_EDGE ( 'NONE', *, *, #24444, .T. ) ;
#25949=ADVANCED_FACE ( 'NONE', ( #3160 ), #18977, .T. ) ;
#25957=VERTEX_POINT ( 'NONE', #5807 ) ;
#25961=DIRECTION ( 'NONE',  ( 0.000000000000000000, 0.000000000000000000, -1.000000000000000000 ) ) ;
#26046=EDGE_LOOP ( 'NONE', ( #36040, #25365, #22880, #39377 ) ) ;
#26196=LINE ( 'NONE', #10327, #13536 ) ;
#26212=EDGE_LOOP ( 'NONE', ( #27234, #34641 ) ) ;
#26262=LINE ( 'NONE', #7111, #39347 ) ;
#26402=CIRCLE ( 'NONE', #39539, 4.357836081054403010 ) ;
#26412=CARTESIAN_POINT ( 'NONE',  ( -70.48694192573870509, 0.1213051481704135875, 5.996540489601009050 ) ) ;
#26456=EDGE_CURVE ( 'NONE', #2282, #6990, #8586, .T. ) ;
#26476=CARTESIAN_POINT ( 'NONE',  ( -70.92837670882107659, 28.72470171467712063, -6.406751979251626317 ) ) ;
#26573=EDGE_LOOP ( 'NONE', ( #21271, #37023, #25666, #202 ) ) ;
#26606=CARTESIAN_POINT ( 'NONE',  ( -69.94741522153590552, -0.5593530815884721896, 5.931425411825930638 ) ) ;
#26807=CARTESIAN_POINT ( 'NONE',  ( -69.98383490720681266, -0.4546002296310912572, 5.937231121521810095 ) ) ;
#26812=EDGE_CURVE ( 'NONE', #5710, #30983, #29094, .T. ) ;
#26860=VECTOR ( 'NONE', #35712, 1000.000000000000000 ) ;
#26903=CARTESIAN_POINT ( 'NONE',  ( -70.92837670882107659, -31.30579396504363388, -4.357836081054403010 ) ) ;
#26919=CARTESIAN_POINT ( 'NONE',  ( -70.31445380653427435, -21.58328887519855854, 5.969244343896258798 ) ) ;
#26938=EDGE_CURVE ( 'NONE', #16289, #38679, #35885, .T. ) ;
#26943=DIRECTION ( 'NONE',  ( 0.000000000000000000, 0.000000000000000000, 1.000000000000000000 ) ) ;
#26954=ADVANCED_FACE ( 'NONE', ( #8049 ), #18343, .T. ) ;
#27004=CARTESIAN_POINT ( 'NONE',  ( -70.07498307583588826, -0.2501102476861906676, 5.951446729975970129 ) ) ;
#27105=CARTESIAN_POINT ( 'NONE',  ( -71.92837670882107659, 28.72470171467712063, 5.916079783099620570 ) ) ;
#27110=CARTESIAN_POINT ( 'NONE',  ( -71.55887904216392315, -21.56717086459383026, 5.979574859000726939 ) ) ;
#27121=CARTESIAN_POINT ( 'NONE',  ( -70.12836265542944147, -21.39718080098120012, 5.947163767836362247 ) ) ;
#27197=FACE_OUTER_BOUND ( 'NONE', #13379, .T. ) ;
#27234=ORIENTED_EDGE ( 'NONE', *, *, #23474, .F. ) ;
#27249=FACE_OUTER_BOUND ( 'NONE', #8350, .T. ) ;
#27325=FACE_OUTER_BOUND ( 'NONE', #28492, .T. ) ;
#27404=CARTESIAN_POINT ( 'NONE',  ( -71.92837670882107659, -0.7434385580723641418, 5.928123921495646265 ) ) ;
#27505=DIRECTION ( 'NONE',  ( -0.8660254037844381525, 0.000000000000000000, 0.5000000000000008882 ) ) ;
#27525=CARTESIAN_POINT ( 'NONE',  ( -69.92837670882107659, -20.82254431570259001, 3.916079783099620126 ) ) ;
#27582=ORIENTED_EDGE ( 'NONE', *, *, #33196, .T. ) ;
#27609=CARTESIAN_POINT ( 'NONE',  ( -70.81198565705318515, 0.2164538760997103128, 3.999856464806924361 ) ) ;
#27655=B_SPLINE_CURVE_WITH_KNOTS ( 'NONE', 3,
 ( #7634, #7233, #19794, #7031, #3972, #29467, #16886, #13611, #19600, #1676 ),
 .UNSPECIFIED., .F., .F.,
 ( 4, 2, 2, 2, 4 ),
 ( 1.084202172485504434E-19, 0.0003915860703966683948, 0.0007831721407933366812, 0.001174758211190004859, 0.001566344281586673146 ),
 .UNSPECIFIED. ) ;
#27665=EDGE_LOOP ( 'NONE', ( #28118, #20, #18944, #11921 ) ) ;
#27739=ADVANCED_FACE ( 'NONE', ( #7434, #35467 ), #23688, .F. ) ;
#27740=DIRECTION ( 'NONE',  ( -0.000000000000000000, 1.000000000000000000, -0.000000000000000000 ) ) ;
#27757=VERTEX_POINT ( 'NONE', #29274 ) ;
#27770=ORIENTED_EDGE ( 'NONE', *, *, #8105, .F. ) ;
#27807=CARTESIAN_POINT ( 'NONE',  ( -71.35621909400492768, 0.1208619214844364048, 3.984726467720987042 ) ) ;
#27812=CARTESIAN_POINT ( 'NONE',  ( -71.72734055786713725, -21.39831690710585477, 5.947291465561956869 ) ) ;
#27921=CARTESIAN_POINT ( 'NONE',  ( -70.14820770166069508, -21.41850222705690143, 5.961650403247820584 ) ) ;
#27926=EDGE_CURVE ( 'NONE', #4011, #9702, #17905, .T. ) ;
#28027=DIRECTION ( 'NONE',  ( 0.000000000000000000, 0.000000000000000000, 1.000000000000000000 ) ) ;
#28058=LINE ( 'NONE', #15088, #13772 ) ;
#28065=DIRECTION ( 'NONE',  ( 0.000000000000000000, 0.000000000000000000, -1.000000000000000000 ) ) ;
#28101=CARTESIAN_POINT ( 'NONE',  ( -64.78958187800138546, -27.85319909218681644, 0.000000000000000000 ) ) ;
#28115=FACE_OUTER_BOUND ( 'NONE', #38053, .T. ) ;
#28118=ORIENTED_EDGE ( 'NONE', *, *, #26938, .F. ) ;
#28168=DIRECTION ( 'NONE',  ( 0.000000000000000000, 0.000000000000000000, -1.000000000000000000 ) ) ;
#28260=ADVANCED_FACE ( 'NONE', ( #18009, #15547 ), #37762, .F. ) ;
#28317=LINE ( 'NONE', #16167, #35524 ) ;
#28372=CARTESIAN_POINT ( 'NONE',  ( -70.92837670882107659, -27.85319909218681644, 0.000000000000000000 ) ) ;
#28438=CARTESIAN_POINT ( 'NONE',  ( -70.92837670882107659, 28.72470171467712063, 0.000000000000000000 ) ) ;
#28492=EDGE_LOOP ( 'NONE', ( #9057, #9797, #22684, #18245 ) ) ;
#28600=CARTESIAN_POINT ( 'NONE',  ( -70.92837670882074974, 0.2169278855384722815, 6.000000000000007994 ) ) ;
#28644=CARTESIAN_POINT ( 'NONE',  ( -71.72837670882105954, -34.30579396504363388, -1.385640646055078307 ) ) ;
#28886=DIRECTION ( 'NONE',  ( -0.000000000000000000, 0.000000000000000000, 1.000000000000000000 ) ) ;
#28916=DIRECTION ( 'NONE',  ( -0.000000000000000000, 1.000000000000000000, 0.000000000000000000 ) ) ;
#28936=DIRECTION ( 'NONE',  ( 0.000000000000000000, -0.7071067811865474617, -0.7071067811865474617 ) ) ;
#28941=EDGE_CURVE ( 'NONE', #33366, #36200, #2563, .T. ) ;
#29021=ORIENTED_EDGE ( 'NONE', *, *, #39294, .F. ) ;
#29032=CARTESIAN_POINT ( 'NONE',  ( -70.92837670882107659, -27.85319909218681644, 0.000000000000000000 ) ) ;
#29088=DIRECTION ( 'NONE',  ( -0.5000000000000008882, 0.000000000000000000, -0.8660254037844382635 ) ) ;
#29094=LINE ( 'NONE', #25401, #20520 ) ;
#29244=ORIENTED_EDGE ( 'NONE', *, *, #35911, .T. ) ;
#29274=CARTESIAN_POINT ( 'NONE',  ( -70.92837670882107659, 26.72470171467712063, -6.406751979251626317 ) ) ;
#29328=AXIS2_PLACEMENT_3D ( 'NONE', #14463, #39582, #23934 ) ;
#29467=CARTESIAN_POINT ( 'NONE',  ( -70.31379738671766688, 0.01634305466338900267, 5.969163363928942090 ) ) ;
#29497=CARTESIAN_POINT ( 'NONE',  ( -69.92837670882107659, -0.7829914368874777431, 3.916079783099610800 ) ) ;
#29530=ADVANCED_FACE ( 'NONE', ( #23263 ), #1643, .T. ) ;
#29536=FACE_OUTER_BOUND ( 'NONE', #26212, .T. ) ;
#29579=AXIS2_PLACEMENT_3D ( 'NONE', #20941, #29802, #14542 ) ;
#29599=CARTESIAN_POINT ( 'NONE',  ( -71.87291851043532631, -21.11138264414386612, 5.937231121521803878 ) ) ;
#29627=DIRECTION ( 'NONE',  ( 0.000000000000000000, 0.000000000000000000, 1.000000000000000000 ) ) ;
#29658=DIRECTION ( 'NONE',  ( -0.000000000000000000, 1.000000000000000000, -0.000000000000000000 ) ) ;
#29768=CARTESIAN_POINT ( 'NONE',  ( -70.92837670882107659, -27.85319909218681644, 0.000000000000000000 ) ) ;
#29790=VERTEX_POINT ( 'NONE', #30316 ) ;
#29802=DIRECTION ( 'NONE',  ( -0.000000000000000000, 1.000000000000000000, -0.000000000000000000 ) ) ;
#29808=CARTESIAN_POINT ( 'NONE',  ( -70.92837670882107659, -27.85319909218681644, 4.357836081054403010 ) ) ;
#29998=ORIENTED_EDGE ( 'NONE', *, *, #17179, .T. ) ;
#30025=CARTESIAN_POINT ( 'NONE',  ( -70.92837670882107659, 26.72470171467712063, 6.406751979251626317 ) ) ;
#30036=CARTESIAN_POINT ( 'NONE',  ( -70.92837670882107659, 28.72470171467712063, 0.000000000000000000 ) ) ;
#30039=ORIENTED_EDGE ( 'NONE', *, *, #11072, .F. ) ;
#30089=EDGE_CURVE ( 'NONE', #8440, #2282, #9648, .T. ) ;
#30103=CARTESIAN_POINT ( 'NONE',  ( -69.92837670882107659, -0.6719362264620037939, 3.916079783099610800 ) ) ;
#30199=CARTESIAN_POINT ( 'NONE',  ( -71.71319929822489314, -21.40271194095481633, 5.960493810635115963 ) ) ;
#30232=FACE_OUTER_BOUND ( 'NONE', #40190, .T. ) ;
#30267=AXIS2_PLACEMENT_3D ( 'NONE', #19620, #29088, #35878 ) ;
#30298=CARTESIAN_POINT ( 'NONE',  ( -70.14355411941724583, -0.1632709328201389365, 3.948449672239096486 ) ) ;
#30316=CARTESIAN_POINT ( 'NONE',  ( -71.92837670882107659, -0.7829914368874776320, 3.916079783099624567 ) ) ;
#30409=CARTESIAN_POINT ( 'NONE',  ( -71.04476776058896803, -21.78243674987466605, 6.011900603202944282 ) ) ;
#30487=DIRECTION ( 'NONE',  ( -0.000000000000000000, 1.000000000000000000, -0.000000000000000000 ) ) ;
#30508=CARTESIAN_POINT ( 'NONE',  ( -71.82557191872977853, -0.3413572496726843264, 5.944584973090449864 ) ) ;
#30618=AXIS2_PLACEMENT_3D ( 'NONE', #23605, #14525, #24208 ) ;
#30670=CARTESIAN_POINT ( 'NONE',  ( -70.92837670882107659, 13.87661300689593880, 0.000000000000000000 ) ) ;
#30719=ORIENTED_EDGE ( 'NONE', *, *, #2526, .T. ) ;
#30744=AXIS2_PLACEMENT_3D ( 'NONE', #35448, #9485, #3553 ) ;
#30748=VECTOR ( 'NONE', #8901, 1000.000000000000000 ) ;
#30754=DIRECTION ( 'NONE',  ( 0.000000000000000000, 0.000000000000000000, 1.000000000000000000 ) ) ;
#30833=ORIENTED_EDGE ( 'NONE', *, *, #30089, .T. ) ;
#30911=EDGE_LOOP ( 'NONE', ( #30039, #38090, #30719, #19395 ) ) ;
#30913=CARTESIAN_POINT ( 'NONE',  ( -70.92837670882107659, 28.72470171467712063, 0.000000000000000000 ) ) ;
#30924=CARTESIAN_POINT ( 'NONE',  ( -71.92602134074772380, -0.7038144147489171498, 5.928523475362950990 ) ) ;
#30983=VERTEX_POINT ( 'NONE', #30025 ) ;
#31038=CARTESIAN_POINT ( 'NONE',  ( -70.50053432363721129, -21.68684479525939324, 5.996770606117007851 ) ) ;
#31039=ORIENTED_EDGE ( 'NONE', *, *, #25812, .T. ) ;
#31124=CARTESIAN_POINT ( 'NONE',  ( -71.54962422038506986, 0.008394241410477492477, 5.980324962551074819 ) ) ;
#31237=STYLED_ITEM('',(#40773),#12327);
#31238=PRODUCT_DEFINITION_CONTEXT ( 'detailed design', #18698, 'design' ) ;
#31279=CARTESIAN_POINT ( 'NONE',  ( -71.92837670882107659, -0.7829914368874778541, 5.916079783099620570 ) ) ;
#31292=DIRECTION ( 'NONE',  ( 0.000000000000000000, 0.000000000000000000, -1.000000000000000000 ) ) ;
#31546=CARTESIAN_POINT ( 'NONE',  ( -69.92844879064466568, -20.91563447912280438, 3.916091967151599462 ) ) ;
#31565=CIRCLE ( 'NONE', #16412, 4.406751979251624540 ) ;
#31786=VECTOR ( 'NONE', #22142, 1000.000000000000000 ) ;
#31897=AXIS2_PLACEMENT_3D ( 'NONE', #16771, #19277, #10406 ) ;
#31925=ORIENTED_EDGE ( 'NONE', *, *, #13852, .F. ) ;
#32018=DIRECTION ( 'NONE',  ( 0.000000000000000000, 0.000000000000000000, 1.000000000000000000 ) ) ;
#32048=AXIS2_PLACEMENT_3D ( 'NONE', #28101, #40656, #18420 ) ;
#32071=VECTOR ( 'NONE', #36336, 1000.000000000000000 ) ;
#32096=DIRECTION ( 'NONE',  ( 0.000000000000000000, -1.000000000000000000, 0.000000000000000000 ) ) ;
#32208=CARTESIAN_POINT ( 'NONE',  ( -70.92837671539291478, 0.2169278822316458022, 3.999987187540717137 ) ) ;
#32256=PRODUCT_CONTEXT ( 'NONE', #11825, 'mechanical' ) ;
#32313=EDGE_LOOP ( 'NONE', ( #29021, #25526, #11242, #14793 ) ) ;
#32392=DIRECTION ( 'NONE',  ( -1.000000000000000000, 0.000000000000000000, -0.000000000000000000 ) ) ;
#32429=( NAMED_UNIT ( * ) SI_UNIT ( $, .STERADIAN. ) SOLID_ANGLE_UNIT ( ) );
#32466=EDGE_LOOP ( 'NONE', ( #8764, #5281, #6490, #37850 ) ) ;
#32533=VECTOR ( 'NONE', #35116, 1000.000000000000000 ) ;
#32598=CARTESIAN_POINT ( 'NONE',  ( -70.29787437547823004, 0.001187990818876110462, 3.967530720604707462 ) ) ;
#32680=AXIS2_PLACEMENT_3D ( 'NONE', #14046, #16722, #23720 ) ;
#32701=CARTESIAN_POINT ( 'NONE',  ( -71.90933819610624766, -21.00662979218648374, 5.931425411825924421 ) ) ;
#32769=CARTESIAN_POINT ( 'NONE',  ( -70.92837670882107659, 13.87661300689593880, 6.000000000000005329 ) ) ;
#32880=CIRCLE ( 'NONE', #29579, 3.784187430299790211 ) ;
#32884=EDGE_CURVE ( 'NONE', #16289, #33366, #15744, .T. ) ;
#32901=CARTESIAN_POINT ( 'NONE',  ( -71.71319929822489314, -21.40271194095481633, 3.948449672239095598 ) ) ;
#33108=VECTOR ( 'NONE', #19057, 1000.000000000000000 ) ;
#33110=EDGE_CURVE ( 'NONE', #38572, #33366, #23676, .T. ) ;
#33142=VERTEX_POINT ( 'NONE', #36847 ) ;
#33196=EDGE_CURVE ( 'NONE', #7083, #16289, #3959, .T. ) ;
#33202=CARTESIAN_POINT ( 'NONE',  ( -70.92837670882107659, -27.85319909218681644, -6.138794830819693793 ) ) ;
#33259=LINE ( 'NONE', #13708, #18163 ) ;
#33274=ORIENTED_EDGE ( 'NONE', *, *, #28941, .F. ) ;
#33285=CYLINDRICAL_SURFACE ( 'NONE', #24638, 3.784187430299790211 ) ;
#33299=EDGE_LOOP ( 'NONE', ( #10628, #3859 ) ) ;
#33366=VERTEX_POINT ( 'NONE', #9 ) ;
#33545=DIRECTION ( 'NONE',  ( 0.8660254037844393737, 0.000000000000000000, 0.4999999999999985567 ) ) ;
#33578=EDGE_CURVE ( 'NONE', #9702, #38572, #2934, .T. ) ;
#33611=CARTESIAN_POINT ( 'NONE',  ( -71.90801809991052096, -0.5528860982213333886, 3.919500413570160990 ) ) ;
#33619=ORIENTED_EDGE ( 'NONE', *, *, #2622, .F. ) ;
#33714=CARTESIAN_POINT ( 'NONE',  ( -70.93014222716664108, -21.78919581838237463, 6.013069300985384835 ) ) ;
#33757=ORIENTED_EDGE ( 'NONE', *, *, #5170, .F. ) ;
#33779=CARTESIAN_POINT ( 'NONE',  ( -71.80203242198795976, -21.28647353953329358, 3.936269516591345052 ) ) ;
#33990=CARTESIAN_POINT ( 'NONE',  ( -71.19182660343213342, -21.78270726315146888, 4.000000000152813762 ) ) ;
#34044=DIRECTION ( 'NONE',  ( 0.000000000000000000, 0.000000000000000000, 1.000000000000000000 ) ) ;
#34050=ORIENTED_EDGE ( 'NONE', *, *, #8105, .T. ) ;
#34110=CIRCLE ( 'NONE', #3874, 6.000000000000005329 ) ;
#34122=CARTESIAN_POINT ( 'NONE',  ( -70.40641634670110705, 0.1089831108692859846, 3.980161455439681806 ) ) ;
#34198=CARTESIAN_POINT ( 'NONE',  ( -71.92837670882107659, -20.78299143688747819, 3.916079783099621014 ) ) ;
#34250=CARTESIAN_POINT ( 'NONE',  ( -70.92837670882107659, -27.85319909218681644, 0.000000000000000000 ) ) ;
#34357=CARTESIAN_POINT ( 'NONE',  ( -70.92837670882107659, 28.72470171467712063, 4.357836081054403010 ) ) ;
#34428=CARTESIAN_POINT ( 'NONE',  ( -71.14735168035940660, 0.1989745095792901375, 6.009053033063231020 ) ) ;
#34527=LINE ( 'NONE', #18849, #38152 ) ;
#34602=ORIENTED_EDGE ( 'NONE', *, *, #2862, .F. ) ;
#34641=ORIENTED_EDGE ( 'NONE', *, *, #22898, .F. ) ;
#34655=CARTESIAN_POINT ( 'NONE',  ( -70.42518057789641261, -21.65701446794189522, 3.980077070345712009 ) ) ;
#34681=CARTESIAN_POINT ( 'NONE',  ( -71.92830462699674854, -0.6503483942891489233, 3.916091967151727804 ) ) ;
#34705=VERTEX_POINT ( 'NONE', #19819 ) ;
#34737=DIRECTION ( 'NONE',  ( -0.000000000000000000, 1.000000000000000000, -0.000000000000000000 ) ) ;
#34871=CARTESIAN_POINT ( 'NONE',  ( -70.92837670882107659, -31.30579396504363388, 0.000000000000000000 ) ) ;
#34919=DIRECTION ( 'NONE',  ( 0.000000000000000000, 0.000000000000000000, 1.000000000000000000 ) ) ;
#35029=CYLINDRICAL_SURFACE ( 'NONE', #14127, 4.357836081054403010 ) ;
#35067=EDGE_CURVE ( 'NONE', #39825, #4011, #2370, .T. ) ;
#35112=CARTESIAN_POINT ( 'NONE',  ( -66.57054062776667536, -31.30579396504363388, 0.000000000000000000 ) ) ;
#35116=DIRECTION ( 'NONE',  ( 0.000000000000000000, 0.000000000000000000, -1.000000000000000000 ) ) ;
#35129=PRODUCT_DEFINITION_SHAPE ( 'NONE', 'NONE',  #21965 ) ;
#35204=CARTESIAN_POINT ( 'NONE',  ( -71.54229961110792146, 0.01730600142359826898, 5.969244343896260574 ) ) ;
#35251=ADVANCED_FACE ( 'NONE', ( #19271 ), #19068, .T. ) ;
#35295=CARTESIAN_POINT ( 'NONE',  ( -69.92837670882107659, 28.72470171467712063, 5.916079783099620570 ) ) ;
#35365=PRODUCT_DEFINITION_FORMATION_WITH_SPECIFIED_SOURCE ( 'ANY', '', #4229, .NOT_KNOWN. ) ;
#35443=CARTESIAN_POINT ( 'NONE',  ( -70.92837670882107659, -23.80776546975053165, -6.000000000000005329 ) ) ;
#35448=CARTESIAN_POINT ( 'NONE',  ( 0.000000000000000000, 0.000000000000000000, 0.000000000000000000 ) ) ;
#35460=CYLINDRICAL_SURFACE ( 'NONE', #7809, 6.000000000000005329 ) ;
#35467=FACE_OUTER_BOUND ( 'NONE', #38290, .T. ) ;
#35524=VECTOR ( 'NONE', #28936, 1000.000000000000114 ) ;
#35597=CARTESIAN_POINT ( 'NONE',  ( -71.36981149190343388, -21.68728802194536698, 3.984496351204982467 ) ) ;
#35615=EDGE_CURVE ( 'NONE', #30983, #27757, #395, .T. ) ;
#35624=DIRECTION ( 'NONE',  ( -0.000000000000000000, 1.000000000000000000, -0.000000000000000000 ) ) ;
#35646=SHAPE_REPRESENTATION_RELATIONSHIP ( 'NONE' , 'NONE' ,  #39290, #17602 ) ;
#35683=CYLINDRICAL_SURFACE ( 'NONE', #13211, 6.000000000000005329 ) ;
#35710=PLANE ( 'NONE',  #5016 ) ;
#35712=DIRECTION ( 'NONE',  ( -0.000000000000000000, 1.000000000000000000, -0.000000000000000000 ) ) ;
#35800=AXIS2_PLACEMENT_3D ( 'NONE', #20405, #10338, #10727 ) ;
#35846=EDGE_CURVE ( 'NONE', #10250, #36200, #26196, .T. ) ;
#35878=DIRECTION ( 'NONE',  ( -0.8660254037844381525, 0.000000000000000000, 0.5000000000000007772 ) ) ;
#35885=LINE ( 'NONE', #10939, #2824 ) ;
#35911=EDGE_CURVE ( 'NONE', #5317, #462, #37864, .T. ) ;
#35987=CARTESIAN_POINT ( 'NONE',  ( -71.87291851043532631, -21.11138264414386612, 3.925186983125783513 ) ) ;
#36039=ADVANCED_FACE ( 'NONE', ( #7486, #923 ), #35710, .F. ) ;
#36040=ORIENTED_EDGE ( 'NONE', *, *, #20042, .T. ) ;
#36078=CIRCLE ( 'NONE', #13052, 6.138794830819693793 ) ;
#36101=VECTOR ( 'NONE', #5426, 1000.000000000000000 ) ;
#36174=AXIS2_PLACEMENT_3D ( 'NONE', #18505, #6, #31292 ) ;
#36200=VERTEX_POINT ( 'NONE', #22948 ) ;
#36223=ORIENTED_EDGE ( 'NONE', *, *, #2622, .T. ) ;
#36242=DIRECTION ( 'NONE',  ( 0.000000000000000000, 0.000000000000000000, -1.000000000000000000 ) ) ;
#36316=CARTESIAN_POINT ( 'NONE',  ( -71.19099899316580604, 0.1905038897469244485, 3.995461420880249470 ) ) ;
#36336=DIRECTION ( 'NONE',  ( -0.000000000000000000, 1.000000000000000000, -0.000000000000000000 ) ) ;
#36346=CARTESIAN_POINT ( 'NONE',  ( -70.92837670882107659, 28.72470171467712063, 4.406751979251624540 ) ) ;
#36382=CARTESIAN_POINT ( 'NONE',  ( -71.92837670882107659, -20.89404664731295114, 5.928123921495630277 ) ) ;
#36486=LINE ( 'NONE', #7874, #39606 ) ;
#36523=AXIS2_PLACEMENT_3D ( 'NONE', #11030, #11434, #21139 ) ;
#36583=CARTESIAN_POINT ( 'NONE',  ( -69.93073207689441517, -20.86216845902604078, 3.916479336966924407 ) ) ;
#36617=ORIENTED_EDGE ( 'NONE', *, *, #27926, .T. ) ;
#36666=CARTESIAN_POINT ( 'NONE',  ( -66.52162472956945294, 28.72470171467712063, 0.000000000000000000 ) ) ;
#36671=CARTESIAN_POINT ( 'NONE',  ( -71.03752578197757828, 0.2110339550563472832, 3.999007124502271804 ) ) ;
#36713=CARTESIAN_POINT ( 'NONE',  ( -71.72694006223731833, -0.1672829062043898751, 3.947339383436517135 ) ) ;
#36751=VERTEX_POINT ( 'NONE', #11114 ) ;
#36784=CARTESIAN_POINT ( 'NONE',  ( -69.98161893566610559, -21.12393755324485412, 3.925045345733725988 ) ) ;
#36807=CARTESIAN_POINT ( 'NONE',  ( -71.92837670882107659, -20.78299143688747819, 3.916079783099621014 ) ) ;
#36847=CARTESIAN_POINT ( 'NONE',  ( -71.72837670882105954, -31.30579396504363388, 1.385640646055090519 ) ) ;
#36879=CARTESIAN_POINT ( 'NONE',  ( -71.92837670882107659, -0.7829914368874768549, 5.928123921495646265 ) ) ;
#36886=CARTESIAN_POINT ( 'NONE',  ( -71.80155306977633245, -21.28742820676846037, 5.936342406970499752 ) ) ;
#36922=LINE ( 'NONE', #37117, #36101 ) ;
#36939=LINE ( 'NONE', #23959, #32071 ) ;
#36986=CARTESIAN_POINT ( 'NONE',  ( -69.94873531773163222, -21.01309677555362398, 3.919500413570160102 ) ) ;
#37023=ORIENTED_EDGE ( 'NONE', *, *, #8570, .T. ) ;
#37117=CARTESIAN_POINT ( 'NONE',  ( -69.32837670882108227, -34.30579396504363388, 1.870248747537495149E-15 ) ) ;
#37249=CARTESIAN_POINT ( 'NONE',  ( -71.92830466161952074, -20.91387172644695980, 3.916091961299410951 ) ) ;
#37283=CARTESIAN_POINT ( 'NONE',  ( -71.92133747557326728, -0.6645477131579885510, 3.917265324091090406 ) ) ;
#37394=CARTESIAN_POINT ( 'NONE',  ( -70.81922763566456069, -21.77701682883130019, 3.999007124502270916 ) ) ;
#37395=UNCERTAINTY_MEASURE_WITH_UNIT (LENGTH_MEASURE( 1.000000000000000082E-05 ), #23354, 'distance_accuracy_value', 'NONE');
#37423=CARTESIAN_POINT ( 'NONE',  ( -71.72837670882105954, -34.30579396504363388, 1.385640646055090519 ) ) ;
#37433=ORIENTED_EDGE ( 'NONE', *, *, #9276, .F. ) ;
#37481=ADVANCED_FACE ( 'NONE', ( #15818 ), #24102, .T. ) ;
#37493=CARTESIAN_POINT ( 'NONE',  ( -70.79671605999898532, -21.78301244779445511, 3.999999999923640193 ) ) ;
#37505=CIRCLE ( 'NONE', #9921, 3.784187430299790211 ) ;
#37540=ADVANCED_FACE ( 'NONE', ( #27249 ), #21289, .T. ) ;
#37636=CARTESIAN_POINT ( 'NONE',  ( -71.92837670882109080, -0.6506956803064269934, 5.916079783099621459 ) ) ;
#37709=VECTOR ( 'NONE', #17316, 1000.000000000000000 ) ;
#37762=PLANE ( 'NONE',  #32048 ) ;
#37775=DIRECTION ( 'NONE',  ( 0.000000000000000000, 0.000000000000000000, 1.000000000000000000 ) ) ;
#37778=ADVANCED_FACE ( 'NONE', ( #38138 ), #3794, .T. ) ;
#37796=EDGE_LOOP ( 'NONE', ( #21264, #98, #29998, #10544 ) ) ;
#37850=ORIENTED_EDGE ( 'NONE', *, *, #6142, .F. ) ;
#37864=CIRCLE ( 'NONE', #8941, 6.000000000000005329 ) ;
#37877=CARTESIAN_POINT ( 'NONE',  ( -71.72837670882105954, -31.30579396504363388, -1.385640646055078307 ) ) ;
#37883=EDGE_LOOP ( 'NONE', ( #11950, #38051, #9899, #2319, #38189, #11296 ) ) ;
#37888=ORIENTED_EDGE ( 'NONE', *, *, #14799, .F. ) ;
#38010=CARTESIAN_POINT ( 'NONE',  ( -70.92837670882107659, 13.87661300689593880, 3.784187430299790211 ) ) ;
#38039=ADVANCED_FACE ( 'NONE', ( #27325 ), #24238, .F. ) ;
#38044=AXIS2_PLACEMENT_3D ( 'NONE', #29768, #11422, #23987 ) ;
#38051=ORIENTED_EDGE ( 'NONE', *, *, #15191, .F. ) ;
#38053=EDGE_LOOP ( 'NONE', ( #6271, #1304, #18647, #40627, #33757, #7567, #6931, #9569 ) ) ;
#38058=CARTESIAN_POINT ( 'NONE',  ( -71.72839076221272592, -0.1688020727937513676, 5.947163767836365800 ) ) ;
#38090=ORIENTED_EDGE ( 'NONE', *, *, #9302, .T. ) ;
#38109=CARTESIAN_POINT ( 'NONE',  ( -70.66575442428671749, -21.75648676341283760, 3.995461420868123170 ) ) ;
#38138=FACE_OUTER_BOUND ( 'NONE', #1574, .T. ) ;
#38152=VECTOR ( 'NONE', #5893, 1000.000000000000114 ) ;
#38170=CARTESIAN_POINT ( 'NONE',  ( -71.72837670882105954, -31.30579396504363388, 1.385640646055090519 ) ) ;
#38189=ORIENTED_EDGE ( 'NONE', *, *, #33110, .T. ) ;
#38270=ORIENTED_EDGE ( 'NONE', *, *, #13488, .T. ) ;
#38290=EDGE_LOOP ( 'NONE', ( #900, #29244 ) ) ;
#38572=VERTEX_POINT ( 'NONE', #8721 ) ;
#38674=EDGE_CURVE ( 'NONE', #40423, #13186, #10548, .T. ) ;
#38679=VERTEX_POINT ( 'NONE', #32208 ) ;
#38785=VERTEX_POINT ( 'NONE', #33202 ) ;
#38941=CARTESIAN_POINT ( 'NONE',  ( -70.59363788503038961, 0.1660198011701667642, 6.003704795174114039 ) ) ;
#38983=ADVANCED_FACE ( 'NONE', ( #17415 ), #24380, .T. ) ;
#39143=CARTESIAN_POINT ( 'NONE',  ( -70.48694192573870509, 0.1213051481704135875, 3.984496351204983355 ) ) ;
#39151=DIRECTION ( 'NONE',  ( -0.000000000000000000, 1.000000000000000000, -0.000000000000000000 ) ) ;
#39250=CARTESIAN_POINT ( 'NONE',  ( -71.92837670882107659, -20.89404664731295114, 3.916079783099609912 ) ) ;
#39290=SHAPE_REPRESENTATION ( 'Triangular punching die', ( #30744 ), #15591 ) ;
#39294=EDGE_CURVE ( 'NONE', #8622, #30983, #33259, .T. ) ;
#39347=VECTOR ( 'NONE', #34737, 1000.000000000000000 ) ;
#39377=ORIENTED_EDGE ( 'NONE', *, *, #6719, .T. ) ;
#39463=CARTESIAN_POINT ( 'NONE',  ( -69.95477047248566294, -21.04545455497950712, 5.920697336060226412 ) ) ;
#39539=AXIS2_PLACEMENT_3D ( 'NONE', #29032, #35624, #29627 ) ;
#39550=CARTESIAN_POINT ( 'NONE',  ( -70.07498307583588826, -0.2501102476861906676, 3.939402591579944435 ) ) ;
#39582=DIRECTION ( 'NONE',  ( -0.000000000000000000, 1.000000000000000000, -0.000000000000000000 ) ) ;
#39606=VECTOR ( 'NONE', #17320, 1000.000000000000114 ) ;
#39660=CARTESIAN_POINT ( 'NONE',  ( -71.46462112523092003, -21.62705418684702252, 3.975988782274377797 ) ) ;
#39671=CARTESIAN_POINT ( 'NONE',  ( -70.66674249470580094, -21.75688355017156184, 5.995522264747396690 ) ) ;
#39691=ADVANCED_FACE ( 'NONE', ( #10748 ), #3215, .T. ) ;
#39731=VERTEX_POINT ( 'NONE', #4201 ) ;
#39733=ORIENTED_EDGE ( 'NONE', *, *, #38674, .F. ) ;
#39755=PLANE ( 'NONE',  #14369 ) ;
#39781=ORIENTED_EDGE ( 'NONE', *, *, #6719, .F. ) ;
#39825=VERTEX_POINT ( 'NONE', #35443 ) ;
#39842=ADVANCED_FACE ( 'NONE', ( #23468 ), #15561, .T. ) ;
#39919=CARTESIAN_POINT ( 'NONE',  ( -70.92837670882107659, -31.30579396504363388, 4.357836081054403010 ) ) ;
#39951=DIRECTION ( 'NONE',  ( -0.000000000000000000, 1.000000000000000000, -0.000000000000000000 ) ) ;
#39967=CARTESIAN_POINT ( 'NONE',  ( -71.87513448197603338, -0.4420453205300980959, 5.937089484129752570 ) ) ;
#40011=CARTESIAN_POINT ( 'NONE',  ( -71.92837670882107659, -20.78299143688747819, 5.916079783099620570 ) ) ;
#40034=EDGE_LOOP ( 'NONE', ( #39733, #21730, #24521, #25063 ) ) ;
#40052=DIRECTION ( 'NONE',  ( -0.000000000000000000, 1.000000000000000000, -0.000000000000000000 ) ) ;
#40077=CARTESIAN_POINT ( 'NONE',  ( -69.94873531773163222, -21.01309677555362398, 5.931544551966180912 ) ) ;
#40166=CARTESIAN_POINT ( 'NONE',  ( -71.03752578197757828, 0.2110339550563472832, 6.011051262898297942 ) ) ;
#40190=EDGE_LOOP ( 'NONE', ( #7276, #16619, #3178, #2543 ) ) ;
#40201=CARTESIAN_POINT ( 'NONE',  ( -69.92837670882107659, 28.72470171467712063, 3.916079783099620126 ) ) ;
#40241=ORIENTED_EDGE ( 'NONE', *, *, #11054, .T. ) ;
#40272=CARTESIAN_POINT ( 'NONE',  ( -70.40039547503687345, -21.63944369480664776, 3.977567636976454768 ) ) ;
#40293=DIRECTION ( 'NONE',  ( 0.000000000000000000, 0.000000000000000000, 1.000000000000000000 ) ) ;
#40365=CARTESIAN_POINT ( 'NONE',  ( -71.05910886569641605, -21.78281089777250301, 5.999999999999995559 ) ) ;
#40379=LINE ( 'NONE', #26476, #3957 ) ;
#40416=EDGE_LOOP ( 'NONE', ( #12767, #40241 ) ) ;
#40423=VERTEX_POINT ( 'NONE', #26903 ) ;
#40533=CARTESIAN_POINT ( 'NONE',  ( -70.92837670882107659, -27.85319909218681644, 6.138794830819693793 ) ) ;
#40559=ORIENTED_EDGE ( 'NONE', *, *, #26938, .T. ) ;
#40563=CARTESIAN_POINT ( 'NONE',  ( -71.90801809991052096, -0.5528860982213333886, 5.931544551966187129 ) ) ;
#40617=EDGE_CURVE ( 'NONE', #7083, #29790, #36939, .T. ) ;
#40627=ORIENTED_EDGE ( 'NONE', *, *, #11832, .F. ) ;
#40656=DIRECTION ( 'NONE',  ( -0.000000000000000000, 1.000000000000000000, 0.000000000000000000 ) ) ;
#40684=CARTESIAN_POINT ( 'NONE',  ( -70.03118149891237465, -21.22462562410226994, 3.932540834694422838 ) ) ;
#40767=COLOUR_RGB('Off White',0.89,0.88,0.83);
#40768=FILL_AREA_STYLE_COLOUR('',#40767);
#40769=FILL_AREA_STYLE('',(#40768));
#40770=SURFACE_STYLE_FILL_AREA(#40769);
#40771=SURFACE_SIDE_STYLE('',(#40770));
#40772=SURFACE_STYLE_USAGE(.BOTH.,#40771);
#40773=PRESENTATION_STYLE_ASSIGNMENT((#40772));
ENDSEC;
END-ISO-10303-21;
